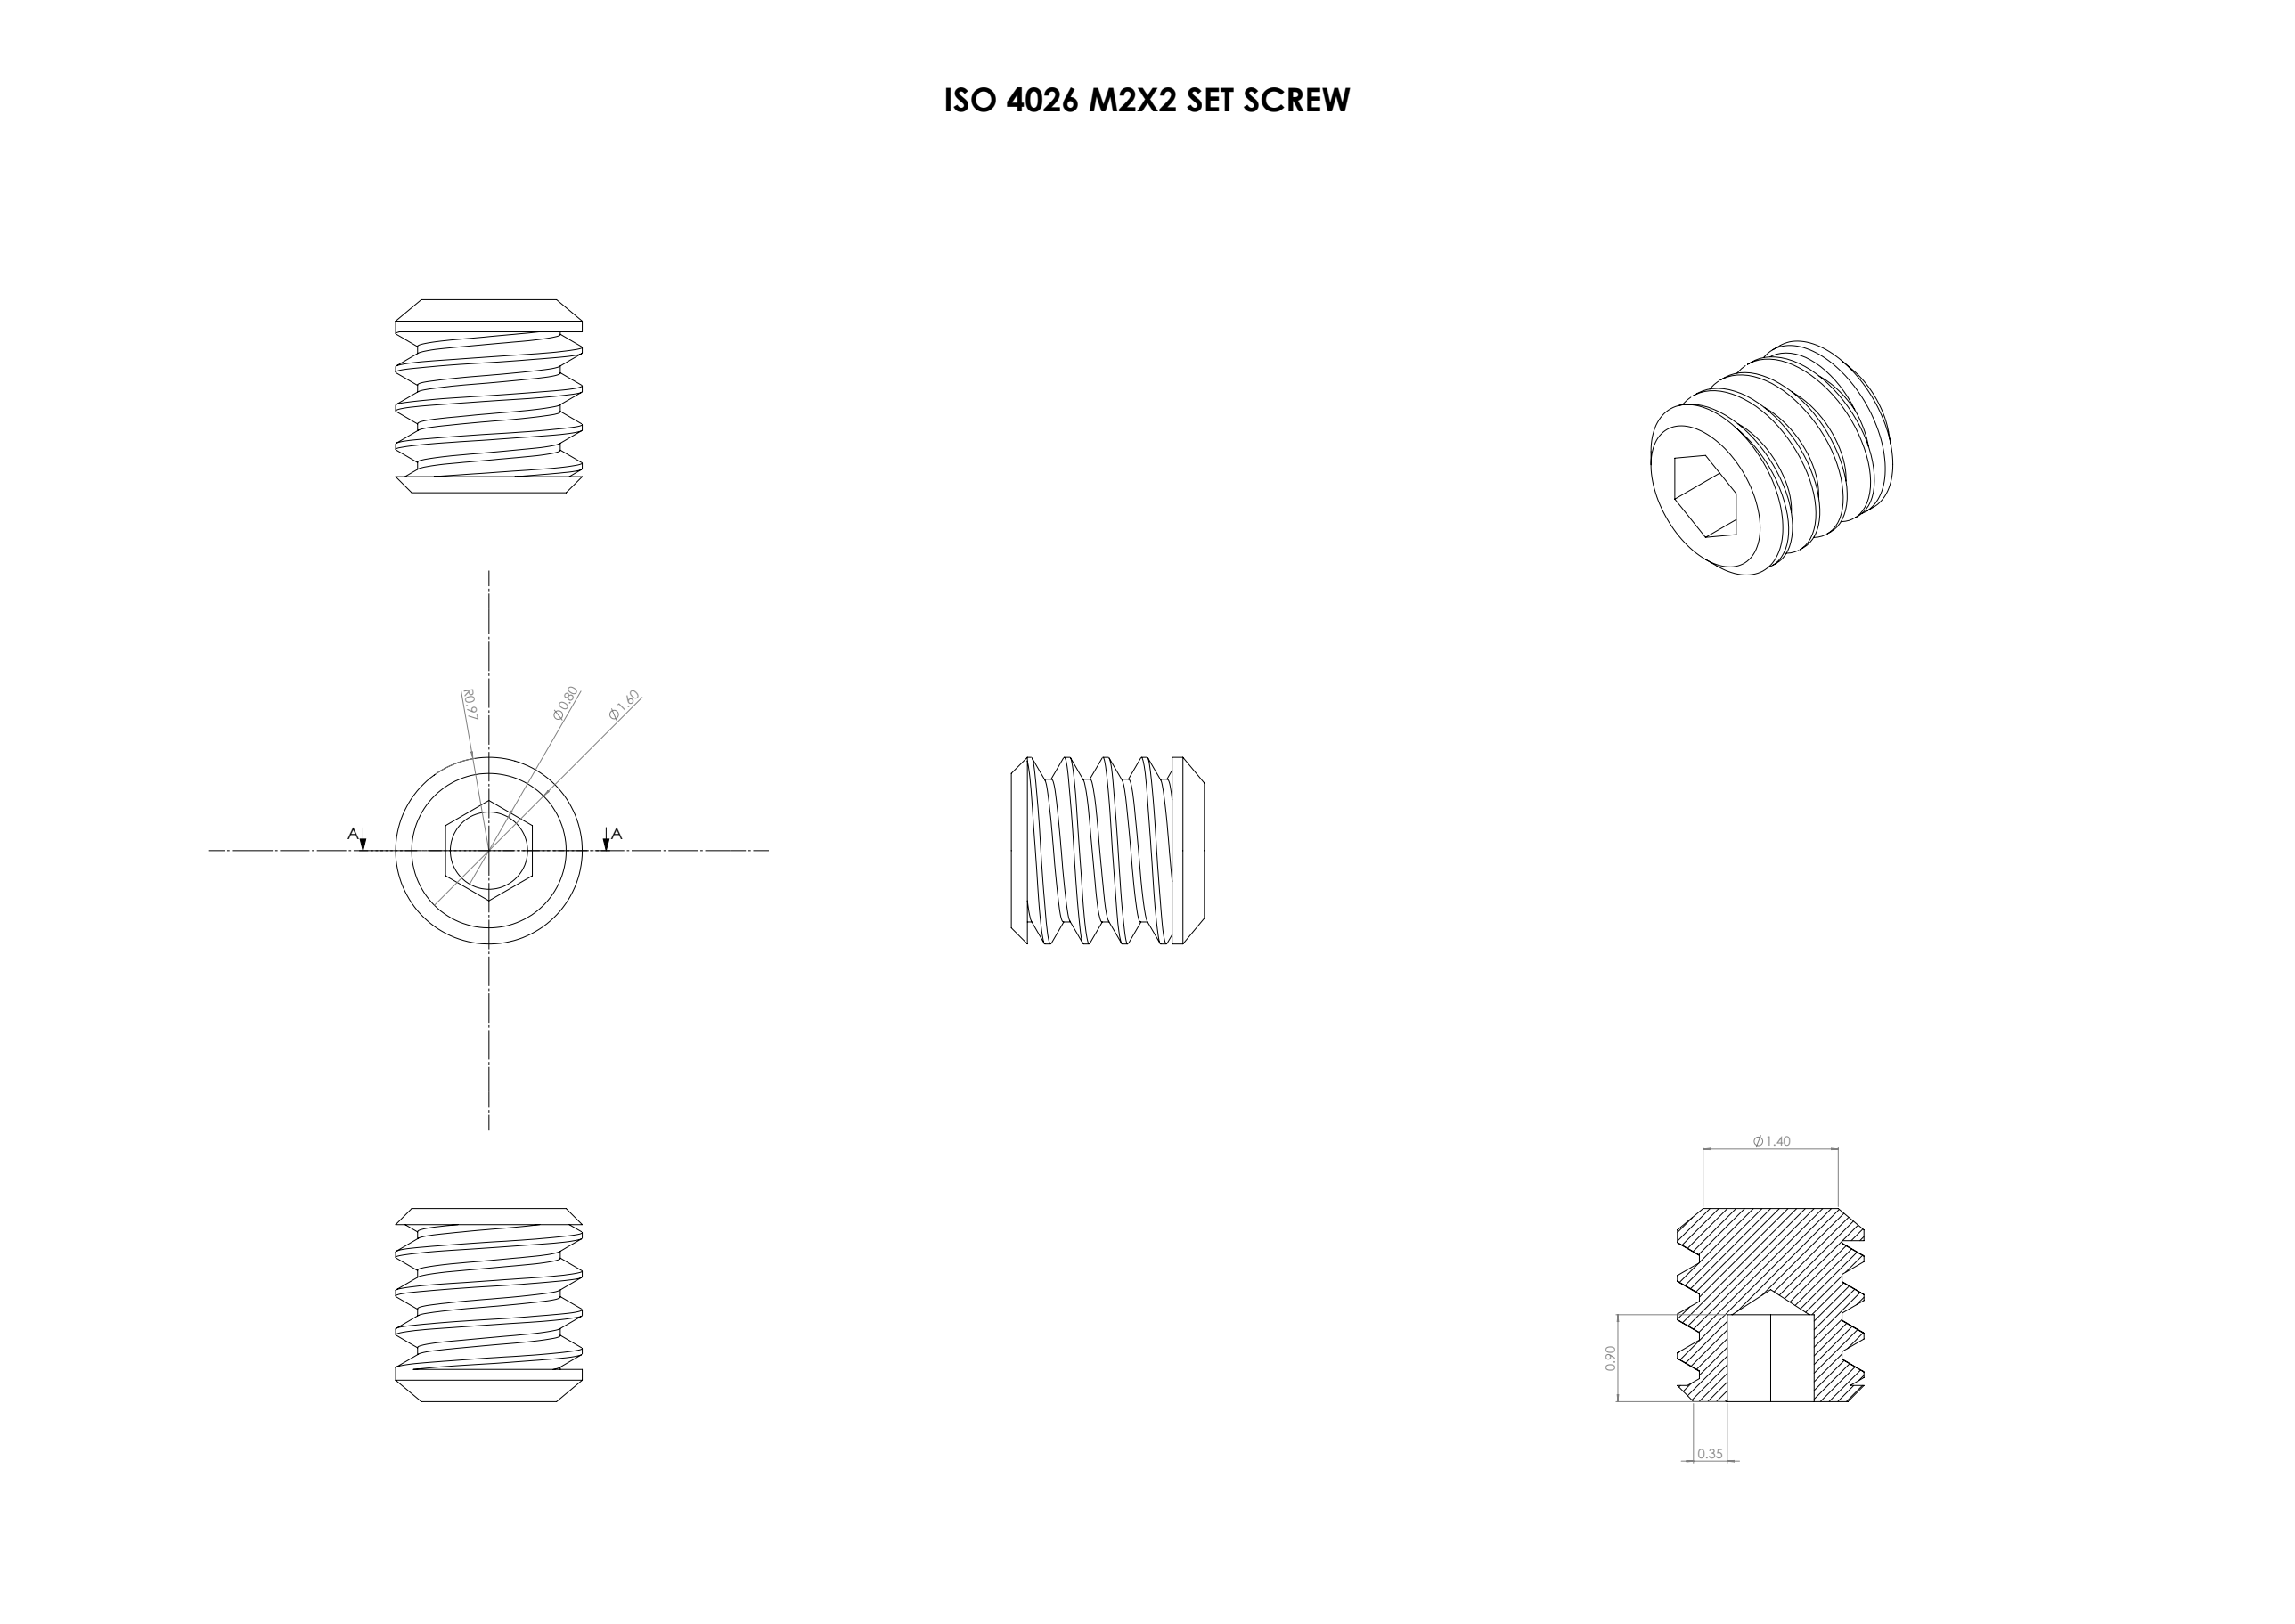
ISO-10303-21;
HEADER;
/* Generated by software containing ST-Developer
 * from STEP Tools, Inc. (www.steptools.com) 
 */

FILE_DESCRIPTION(
/* description */ (''),
/* implementation_level */ '2;1');

FILE_NAME(
/* name */ '20_ISO_4026_M2x2_Set_Screw.step',
/* time_stamp */ '2026-10-19T23:00:43-07:00',
/* author */ (''),
/* organization */ (''),
/* preprocessor_version */ 'ST-DEVELOPER v20.2',
/* originating_system */ 'Autodesk Translation Framework v15.15.0.0',
/* authorisation */ '');

FILE_SCHEMA (('AUTOMOTIVE_DESIGN { 1 0 10303 214 3 1 1 }'));
ENDSEC;

DATA;
#10=MECHANICAL_DESIGN_GEOMETRIC_PRESENTATION_REPRESENTATION('',(#1009),#55002);
#470=B_SPLINE_SURFACE_WITH_KNOTS('',3,3,((#38097,#38098,#38099,#38100,#38101,
#38102,#38103,#38104,#38105,#38106,#38107,#38108,#38109,#38110,#38111,#38112,
#38113,#38114,#38115,#38116,#38117,#38118,#38119,#38120,#38121,#38122,#38123,
#38124,#38125),(#38126,#38127,#38128,#38129,#38130,#38131,#38132,#38133,
#38134,#38135,#38136,#38137,#38138,#38139,#38140,#38141,#38142,#38143,#38144,
#38145,#38146,#38147,#38148,#38149,#38150,#38151,#38152,#38153,#38154),
(#38155,#38156,#38157,#38158,#38159,#38160,#38161,#38162,#38163,#38164,
#38165,#38166,#38167,#38168,#38169,#38170,#38171,#38172,#38173,#38174,#38175,
#38176,#38177,#38178,#38179,#38180,#38181,#38182,#38183),(#38184,#38185,
#38186,#38187,#38188,#38189,#38190,#38191,#38192,#38193,#38194,#38195,#38196,
#38197,#38198,#38199,#38200,#38201,#38202,#38203,#38204,#38205,#38206,#38207,
#38208,#38209,#38210,#38211,#38212)),.UNSPECIFIED.,.F.,.F.,.F.,(4,4),(4,
1,1,1,1,1,1,1,1,1,1,1,1,1,1,1,1,1,1,1,1,1,1,1,1,1,4),(0.,0.0262983047615875),
(10.0522207760382,11.0378903501899,12.0235599243416,13.0092294984934,13.9948990726451,
14.9805686467968,15.9662382209486,16.9519077951003,17.937577369252,18.9232469434038,
19.9089165175555,20.8945860917073,21.880255665859,22.8659252400107,23.8515948141625,
24.8372643883142,25.8229339624659,26.8086035366177,27.7942731107694,28.7799426849212,
29.7656122590729,30.7512818332246,31.7369514073764,32.7226209815281,33.7082905556798,
34.6939601298316,35.6796297039833),.UNSPECIFIED.);
#471=B_SPLINE_SURFACE_WITH_KNOTS('',3,3,((#38342,#38343,#38344,#38345,#38346,
#38347,#38348,#38349,#38350,#38351,#38352,#38353,#38354,#38355,#38356,#38357,
#38358,#38359,#38360,#38361,#38362,#38363,#38364,#38365,#38366,#38367,#38368,
#38369,#38370),(#38371,#38372,#38373,#38374,#38375,#38376,#38377,#38378,
#38379,#38380,#38381,#38382,#38383,#38384,#38385,#38386,#38387,#38388,#38389,
#38390,#38391,#38392,#38393,#38394,#38395,#38396,#38397,#38398,#38399),
(#38400,#38401,#38402,#38403,#38404,#38405,#38406,#38407,#38408,#38409,
#38410,#38411,#38412,#38413,#38414,#38415,#38416,#38417,#38418,#38419,#38420,
#38421,#38422,#38423,#38424,#38425,#38426,#38427,#38428),(#38429,#38430,
#38431,#38432,#38433,#38434,#38435,#38436,#38437,#38438,#38439,#38440,#38441,
#38442,#38443,#38444,#38445,#38446,#38447,#38448,#38449,#38450,#38451,#38452,
#38453,#38454,#38455,#38456,#38457)),.UNSPECIFIED.,.F.,.F.,.F.,(4,4),(4,
1,1,1,1,1,1,1,1,1,1,1,1,1,1,1,1,1,1,1,1,1,1,1,1,1,4),(0.,0.0262983047615875),
(13.3593226216143,14.3449921957661,15.3306617699178,16.3163313440695,17.3020009182213,
18.287670492373,19.2733400665247,20.2590096406765,21.2446792148282,22.23034878898,
23.2160183631317,24.2016879372834,25.1873575114352,26.1730270855869,27.1586966597386,
28.1443662338904,29.1300358080421,30.1157053821939,31.1013749563456,32.0870445304973,
33.0727141046491,34.0583836788008,35.0440532529525,36.0297228271043,37.015392401256,
38.0010619754078,38.9867315495595),.UNSPECIFIED.);
#505=B_SPLINE_CURVE_WITH_KNOTS('',3,(#37754,#37755,#37756,#37757,#37758,
#37759,#37760,#37761,#37762,#37763,#37764,#37765,#37766,#37767,#37768,#37769,
#37770,#37771,#37772,#37773,#37774,#37775),.UNSPECIFIED.,.F.,.F.,(4,3,3,
3,3,3,3,4),(-8.63182595351423,-7.8853565932139,-6.89968701906216,-5.91401744491043,
-4.92834787075869,-3.94267829660695,-2.95700872245521,-2.34864064633464),
 .UNSPECIFIED.);
#506=B_SPLINE_CURVE_WITH_KNOTS('',3,(#37780,#37781,#37782,#37783),
 .UNSPECIFIED.,.F.,.F.,(4,4),(-2.34864064633464,-2.06546402602172),
 .UNSPECIFIED.);
#507=B_SPLINE_CURVE_WITH_KNOTS('',3,(#37786,#37787,#37788,#37789,#37790,
#37791,#37792,#37793,#37794,#37795,#37796,#37797,#37798,#37799,#37800,#37801,
#37802,#37803,#37804),.UNSPECIFIED.,.F.,.F.,(4,3,3,3,3,3,4),(0.,0.985669574151735,
1.97133914830348,2.95700872245521,3.94267829660695,4.92834787075869,5.65574249191081),
 .UNSPECIFIED.);
#508=B_SPLINE_CURVE_WITH_KNOTS('',3,(#37809,#37810,#37811,#37812,#37813,
#37814,#37815,#37816,#37817,#37818,#37819,#37820,#37821,#37822,#37823,#37824,
#37825,#37826,#37827,#37828,#37829,#37830,#37831,#37832,#37833),
 .UNSPECIFIED.,.F.,.F.,(4,3,3,3,3,3,3,3,4),(-14.9150112606938,-14.7850436122761,
-13.7993740381243,-12.8137044639726,-11.8280348898208,-10.8423653156691,
-9.85669574151737,-8.87102616736564,-8.63182595351423),.UNSPECIFIED.);
#509=B_SPLINE_CURVE_WITH_KNOTS('',3,(#37834,#37835,#37836,#37837,#37838,
#37839,#37840,#37841,#37842,#37843,#37844,#37845,#37846,#37847,#37848,#37849,
#37850,#37851,#37852,#37853,#37854,#37855,#37856,#37857,#37858),
 .UNSPECIFIED.,.F.,.F.,(4,3,3,3,3,3,3,3,4),(5.65574249191081,5.91401744491043,
6.89968701906216,7.8853565932139,8.87102616736564,9.85669574151738,10.8423653156691,
11.8280348898208,11.9389277990904),.UNSPECIFIED.);
#510=B_SPLINE_CURVE_WITH_KNOTS('',3,(#37863,#37864,#37865,#37866,#37867,
#37868,#37869,#37870,#37871,#37872,#37873,#37874,#37875,#37876,#37877,#37878,
#37879,#37880,#37881,#37882,#37883,#37884),.UNSPECIFIED.,.F.,.F.,(4,3,3,
3,3,3,3,4),(-21.1981965678734,-20.6990610571865,-19.7133914830348,-18.727721908883,
-17.7420523347313,-16.7563827605795,-15.7707131864278,-14.9150112606938),
 .UNSPECIFIED.);
#511=B_SPLINE_CURVE_WITH_KNOTS('',3,(#37885,#37886,#37887,#37888,#37889,
#37890,#37891,#37892,#37893,#37894,#37895,#37896,#37897,#37898,#37899,#37900,
#37901,#37902,#37903,#37904,#37905,#37906),.UNSPECIFIED.,.F.,.F.,(4,3,3,
3,3,3,3,4),(11.9389277990904,12.8137044639726,13.7993740381243,14.7850436122761,
15.7707131864278,16.7563827605795,17.7420523347313,18.22211310627),
 .UNSPECIFIED.);
#512=B_SPLINE_CURVE_WITH_KNOTS('',3,(#37912,#37913,#37914,#37915,#37916,
#37917),.UNSPECIFIED.,.F.,.F.,(4,1,1,4),(34.5575191894877,35.0440532529525,
36.0297228271043,36.9212675235378),.UNSPECIFIED.);
#513=B_SPLINE_CURVE_WITH_KNOTS('',3,(#37920,#37921,#37922,#37923,#37924),
 .UNSPECIFIED.,.F.,.F.,(4,1,4),(34.5575191894877,34.6939601298316,35.6796297039833),
 .UNSPECIFIED.);
#514=B_SPLINE_CURVE_WITH_KNOTS('',3,(#37929,#37930,#37931,#37932,#37933,
#37934,#37935,#37936,#37937,#37938),.UNSPECIFIED.,.F.,.F.,(4,1,1,1,1,1,
1,4),(28.2743338823081,29.1300358080421,30.1157053821939,31.1013749563456,
32.0870445304973,33.0727141046491,34.0583836788008,34.5575191894877),
 .UNSPECIFIED.);
#515=B_SPLINE_CURVE_WITH_KNOTS('',3,(#37939,#37940,#37941,#37942,#37943,
#37944,#37945,#37946,#37947,#37948),.UNSPECIFIED.,.F.,.F.,(4,1,1,1,1,1,
1,4),(28.2743338823081,28.7799426849212,29.7656122590729,30.7512818332246,
31.7369514073764,32.7226209815281,33.7082905556798,34.5575191894877),
 .UNSPECIFIED.);
#516=B_SPLINE_CURVE_WITH_KNOTS('',3,(#37953,#37954,#37955,#37956,#37957,
#37958,#37959,#37960,#37961,#37962,#37963),.UNSPECIFIED.,.F.,.F.,(4,1,1,
1,1,1,1,1,4),(21.9911485751285,22.23034878898,23.2160183631317,24.2016879372834,
25.1873575114352,26.1730270855869,27.1586966597386,28.1443662338904,28.2743338823081),
 .UNSPECIFIED.);
#517=B_SPLINE_CURVE_WITH_KNOTS('',3,(#37964,#37965,#37966,#37967,#37968,
#37969,#37970,#37971,#37972,#37973),.UNSPECIFIED.,.F.,.F.,(4,1,1,1,1,1,
1,4),(21.9911485751285,22.8659252400107,23.8515948141625,24.8372643883142,
25.8229339624659,26.8086035366177,27.7942731107694,28.2743338823081),
 .UNSPECIFIED.);
#518=B_SPLINE_CURVE_WITH_KNOTS('',3,(#37978,#37979,#37980,#37981,#37982,
#37983,#37984,#37985,#37986,#37987),.UNSPECIFIED.,.F.,.F.,(4,1,1,1,1,1,
1,4),(15.707963267949,16.3163313440695,17.3020009182213,18.287670492373,
19.2733400665247,20.2590096406765,21.2446792148282,21.9911485751285),
 .UNSPECIFIED.);
#519=B_SPLINE_CURVE_WITH_KNOTS('',3,(#37988,#37989,#37990,#37991,#37992,
#37993,#37994,#37995,#37996,#37997,#37998),.UNSPECIFIED.,.F.,.F.,(4,1,1,
1,1,1,1,1,4),(15.707963267949,15.9662382209486,16.9519077951003,17.937577369252,
18.9232469434038,19.9089165175555,20.8945860917073,21.880255665859,21.9911485751285),
 .UNSPECIFIED.);
#520=B_SPLINE_CURVE_WITH_KNOTS('',3,(#38001,#38002,#38003,#38004,#38005,
#38006,#38007,#38008,#38009,#38010,#38011,#38012,#38013,#38014,#38015,#38016,
#38017,#38018,#38019,#38020,#38021,#38022,#38023,#38024,#38025,#38026,#38027,
#38028,#38029,#38030,#38031,#38032,#38033,#38034,#38035,#38036,#38037,#38038,
#38039,#38040,#38041,#38042,#38043,#38044,#38045,#38046),.UNSPECIFIED.,
 .F.,.F.,(4,3,3,3,3,3,3,3,3,3,3,3,3,3,3,4),(-0.178587760439503,-0.171463223481926,
-0.158469202239697,-0.149838461616654,-0.140115954947833,-0.131832290711792,
-0.111519735101834,-0.104220668242419,-0.0909951576576451,-0.0752259129616406,
-0.0672217662272291,-0.0504163246704218,-0.0371902256154733,-0.0290084673554581,
-0.00644509207244406,0.),.UNSPECIFIED.);
#521=B_SPLINE_CURVE_WITH_KNOTS('',3,(#38051,#38052,#38053,#38054,#38055,
#38056,#38057,#38058,#38059,#38060,#38061,#38062,#38063,#38064,#38065,#38066,
#38067,#38068,#38069,#38070,#38071,#38072,#38073,#38074,#38075,#38076,#38077,
#38078,#38079,#38080,#38081,#38082,#38083,#38084,#38085,#38086,#38087,#38088,
#38089,#38090,#38091,#38092,#38093,#38094,#38095,#38096),.UNSPECIFIED.,
 .F.,.F.,(4,3,3,3,3,3,3,3,3,3,3,3,3,3,3,4),(-0.177567088092161,-0.168491849215037,
-0.152129281927587,-0.143009688907872,-0.128326089911933,-0.120351006519644,
-0.0990535795520566,-0.087638613810708,-0.079080103543658,-0.064425434388532,
-0.0552021544374827,-0.041401615828112,-0.0308502855955504,-0.0238678565643904,
-0.00551137719623127,0.),.UNSPECIFIED.);
#522=B_SPLINE_CURVE_WITH_KNOTS('',3,(#38213,#38214,#38215,#38216,#38217,
#38218,#38219,#38220,#38221,#38222,#38223,#38224,#38225,#38226,#38227,#38228,
#38229,#38230,#38231),.UNSPECIFIED.,.F.,.F.,(4,3,3,3,3,3,4),(18.22211310627,
18.727721908883,19.7133914830347,20.6990610571865,21.6847306313382,22.67040020549,
23.5619449019235),.UNSPECIFIED.);
#523=B_SPLINE_CURVE_WITH_KNOTS('',3,(#38233,#38234,#38235,#38236,#38237,
#38238,#38239,#38240,#38241,#38242,#38243,#38244,#38245,#38246,#38247,#38248,
#38249,#38250,#38251,#38252,#38253,#38254,#38255,#38256,#38257,#38258,#38259,
#38260,#38261,#38262,#38263,#38264,#38265,#38266,#38267,#38268,#38269,#38270,
#38271,#38272,#38273,#38274,#38275,#38276,#38277,#38278),.UNSPECIFIED.,
 .F.,.F.,(4,3,3,3,3,3,3,3,3,3,3,3,3,3,3,4),(-0.178587760439501,-0.171463223481924,
-0.158469220396003,-0.149838461060004,-0.140115983264454,-0.131832291484538,
-0.11151973540878,-0.104220666177739,-0.0909951576576466,-0.0752259249257156,
-0.0672217660243099,-0.0504163245182324,-0.0371902270455756,-0.0290084696776603,
-0.00644510100322751,0.),.UNSPECIFIED.);
#524=B_SPLINE_CURVE_WITH_KNOTS('',3,(#38279,#38280,#38281,#38282,#38283,
#38284,#38285),.UNSPECIFIED.,.F.,.F.,(4,1,1,1,4),(12.1176848020599,13.0092294984934,
13.9948990726451,14.9805686467968,15.707963267949),.UNSPECIFIED.);
#525=B_SPLINE_CURVE_WITH_KNOTS('',3,(#38288,#38289,#38290,#38291,#38292,
#38293,#38294,#38295,#38296,#38297,#38298,#38299,#38300,#38301,#38302,#38303,
#38304,#38305,#38306,#38307,#38308,#38309,#38310,#38311,#38312,#38313,#38314,
#38315,#38316,#38317,#38318,#38319,#38320,#38321,#38322,#38323,#38324,#38325,
#38326,#38327,#38328,#38329,#38330,#38331,#38332,#38333),.UNSPECIFIED.,
 .F.,.F.,(4,3,3,3,3,3,3,3,3,3,3,3,3,3,3,4),(-0.177567088092159,-0.168491849215035,
-0.152129287596336,-0.143009693943577,-0.128326090026494,-0.120351011600958,
-0.0990535966185752,-0.087638608675612,-0.0790801035436585,-0.0644254494454798,
-0.0552021579381271,-0.0414016184535953,-0.0308502860822931,-0.0238678558967309,
-0.00551135674322404,0.),.UNSPECIFIED.);
#526=B_SPLINE_CURVE_WITH_KNOTS('',3,(#38336,#38337,#38338,#38339,#38340,
#38341),.UNSPECIFIED.,.F.,.F.,(4,1,1,4),(13.3593226216143,14.3449921957661,
15.3306617699178,15.707963267949),.UNSPECIFIED.);
#527=B_SPLINE_CURVE_WITH_KNOTS('',3,(#38458,#38459,#38460,#38461,#38462,
#38463,#38464,#38465,#38466,#38467,#38468,#38469,#38470,#38471,#38472,#38473),
 .UNSPECIFIED.,.F.,.F.,(4,3,3,3,3,4),(-25.6274089279452,-24.6417393537934,
-23.6560697796417,-22.67040020549,-21.6847306313382,-21.1981965678734),
 .UNSPECIFIED.);
#969=SHAPE_REPRESENTATION_RELATIONSHIP('SRR','None',#55117,#989);
#989=ADVANCED_BREP_SHAPE_REPRESENTATION('',(#1029),#54995);
#1009=STYLED_ITEM('',(#55393),#1029);
#1029=MANIFOLD_SOLID_BREP('Set Screw M2x2',#24542);
#1259=FACE_BOUND('',#4702,.T.);
#1260=FACE_BOUND('',#4707,.T.);
#1537=PLANE('',#26162);
#1538=PLANE('',#26165);
#1539=PLANE('',#26172);
#1540=PLANE('',#26173);
#1541=PLANE('',#26174);
#1542=PLANE('',#26175);
#1543=PLANE('',#26176);
#1544=PLANE('',#26177);
#1545=PLANE('',#26178);
#1546=PLANE('',#26179);
#1547=PLANE('',#26184);
#2193=CYLINDRICAL_SURFACE('',#26152,0.096675);
#2194=CYLINDRICAL_SURFACE('',#26155,0.096675);
#2195=CYLINDRICAL_SURFACE('',#26156,0.096675);
#2196=CYLINDRICAL_SURFACE('',#26157,0.0739);
#2197=CYLINDRICAL_SURFACE('',#26159,0.0739);
#2198=CYLINDRICAL_SURFACE('',#26160,0.0739);
#2199=CYLINDRICAL_SURFACE('',#26161,0.0739);
#2200=CYLINDRICAL_SURFACE('',#26167,0.0739);
#2201=CYLINDRICAL_SURFACE('',#26168,0.096675);
#3094=FACE_OUTER_BOUND('',#4681,.T.);
#3095=FACE_OUTER_BOUND('',#4682,.T.);
#3096=FACE_OUTER_BOUND('',#4683,.T.);
#3097=FACE_OUTER_BOUND('',#4684,.T.);
#3098=FACE_OUTER_BOUND('',#4685,.T.);
#3099=FACE_OUTER_BOUND('',#4686,.T.);
#3100=FACE_OUTER_BOUND('',#4687,.T.);
#3101=FACE_OUTER_BOUND('',#4688,.T.);
#3102=FACE_OUTER_BOUND('',#4689,.T.);
#3103=FACE_OUTER_BOUND('',#4690,.T.);
#3104=FACE_OUTER_BOUND('',#4691,.T.);
#3105=FACE_OUTER_BOUND('',#4692,.T.);
#3106=FACE_OUTER_BOUND('',#4693,.T.);
#3107=FACE_OUTER_BOUND('',#4694,.T.);
#3108=FACE_OUTER_BOUND('',#4695,.T.);
#3109=FACE_OUTER_BOUND('',#4696,.T.);
#3110=FACE_OUTER_BOUND('',#4697,.T.);
#3111=FACE_OUTER_BOUND('',#4698,.T.);
#3112=FACE_OUTER_BOUND('',#4699,.T.);
#3113=FACE_OUTER_BOUND('',#4700,.T.);
#3114=FACE_OUTER_BOUND('',#4701,.T.);
#3115=FACE_OUTER_BOUND('',#4703,.T.);
#3116=FACE_OUTER_BOUND('',#4704,.T.);
#3117=FACE_OUTER_BOUND('',#4705,.T.);
#3118=FACE_OUTER_BOUND('',#4706,.T.);
#4681=EDGE_LOOP('',(#19074,#19075,#19076,#19077,#19078,#19079,#19080,#19081));
#4682=EDGE_LOOP('',(#19082,#19083,#19084,#19085));
#4683=EDGE_LOOP('',(#19086,#19087,#19088,#19089));
#4684=EDGE_LOOP('',(#19090,#19091,#19092,#19093));
#4685=EDGE_LOOP('',(#19094,#19095,#19096,#19097));
#4686=EDGE_LOOP('',(#19098,#19099,#19100,#19101));
#4687=EDGE_LOOP('',(#19102,#19103,#19104,#19105));
#4688=EDGE_LOOP('',(#19106,#19107,#19108,#19109,#19110));
#4689=EDGE_LOOP('',(#19111,#19112,#19113,#19114,#19115,#19116,#19117,#19118,
#19119,#19120,#19121));
#4690=EDGE_LOOP('',(#19122,#19123,#19124,#19125));
#4691=EDGE_LOOP('',(#19126,#19127,#19128,#19129));
#4692=EDGE_LOOP('',(#19130,#19131,#19132,#19133,#19134,#19135,#19136,#19137,
#19138,#19139,#19140,#19141));
#4693=EDGE_LOOP('',(#19142,#19143,#19144,#19145));
#4694=EDGE_LOOP('',(#19146,#19147,#19148));
#4695=EDGE_LOOP('',(#19149,#19150,#19151,#19152));
#4696=EDGE_LOOP('',(#19153,#19154,#19155,#19156));
#4697=EDGE_LOOP('',(#19157,#19158,#19159,#19160));
#4698=EDGE_LOOP('',(#19161,#19162,#19163,#19164));
#4699=EDGE_LOOP('',(#19165,#19166,#19167,#19168));
#4700=EDGE_LOOP('',(#19169,#19170,#19171,#19172));
#4701=EDGE_LOOP('',(#19173,#19174,#19175,#19176,#19177,#19178));
#4702=EDGE_LOOP('',(#19179));
#4703=EDGE_LOOP('',(#19180));
#4704=EDGE_LOOP('',(#19181,#19182,#19183,#19184));
#4705=EDGE_LOOP('',(#19185,#19186,#19187,#19188,#19189,#19190));
#4706=EDGE_LOOP('',(#19191));
#4707=EDGE_LOOP('',(#19192,#19193,#19194,#19195,#19196,#19197));
#6265=LINE('',#37752,#8086);
#6266=LINE('',#37777,#8087);
#6267=LINE('',#37808,#8088);
#6268=LINE('',#37862,#8089);
#6269=LINE('',#37910,#8090);
#6270=LINE('',#37928,#8091);
#6271=LINE('',#37952,#8092);
#6272=LINE('',#37977,#8093);
#6273=LINE('',#38479,#8094);
#6274=LINE('',#38484,#8095);
#6275=LINE('',#38486,#8096);
#6276=LINE('',#38488,#8097);
#6277=LINE('',#38489,#8098);
#6278=LINE('',#38492,#8099);
#6279=LINE('',#38494,#8100);
#6280=LINE('',#38495,#8101);
#6281=LINE('',#38498,#8102);
#6282=LINE('',#38500,#8103);
#6283=LINE('',#38501,#8104);
#6284=LINE('',#38504,#8105);
#6285=LINE('',#38506,#8106);
#6286=LINE('',#38507,#8107);
#6287=LINE('',#38510,#8108);
#6288=LINE('',#38512,#8109);
#6289=LINE('',#38513,#8110);
#6290=LINE('',#38515,#8111);
#6291=LINE('',#38516,#8112);
#6292=LINE('',#38522,#8113);
#6293=LINE('',#38526,#8114);
#8086=VECTOR('',#30847,0.1);
#8087=VECTOR('',#30848,0.1);
#8088=VECTOR('',#30855,0.1);
#8089=VECTOR('',#30858,0.1);
#8090=VECTOR('',#30861,0.0739);
#8091=VECTOR('',#30866,0.0739);
#8092=VECTOR('',#30869,0.0739);
#8093=VECTOR('',#30872,0.0739);
#8094=VECTOR('',#30891,0.0207846096908265);
#8095=VECTOR('',#30896,1.);
#8096=VECTOR('',#30897,1.);
#8097=VECTOR('',#30898,1.);
#8098=VECTOR('',#30899,1.);
#8099=VECTOR('',#30902,1.);
#8100=VECTOR('',#30903,1.);
#8101=VECTOR('',#30904,1.);
#8102=VECTOR('',#30907,1.);
#8103=VECTOR('',#30908,1.);
#8104=VECTOR('',#30909,1.);
#8105=VECTOR('',#30912,1.);
#8106=VECTOR('',#30913,1.);
#8107=VECTOR('',#30914,1.);
#8108=VECTOR('',#30917,1.);
#8109=VECTOR('',#30918,1.);
#8110=VECTOR('',#30919,1.);
#8111=VECTOR('',#30922,1.);
#8112=VECTOR('',#30923,1.);
#8113=VECTOR('',#30932,0.085);
#8114=VECTOR('',#30937,0.09);
#9710=CIRCLE('',#26153,0.096675);
#9711=CIRCLE('',#26154,0.096675);
#9712=CIRCLE('',#26158,0.0739);
#9713=CIRCLE('',#26163,0.096675);
#9714=CIRCLE('',#26164,0.096675);
#9715=CIRCLE('',#26166,0.0739);
#9716=CIRCLE('',#26169,0.096675);
#9717=CIRCLE('',#26171,0.0400285208940887);
#9718=CIRCLE('',#26180,0.07);
#9719=CIRCLE('',#26183,0.08);
#11061=VERTEX_POINT('',#37750);
#11062=VERTEX_POINT('',#37751);
#11063=VERTEX_POINT('',#37753);
#11064=VERTEX_POINT('',#37776);
#11065=VERTEX_POINT('',#37779);
#11066=VERTEX_POINT('',#37784);
#11067=VERTEX_POINT('',#37806);
#11068=VERTEX_POINT('',#37807);
#11069=VERTEX_POINT('',#37860);
#11070=VERTEX_POINT('',#37861);
#11071=VERTEX_POINT('',#37908);
#11072=VERTEX_POINT('',#37909);
#11073=VERTEX_POINT('',#37911);
#11074=VERTEX_POINT('',#37918);
#11075=VERTEX_POINT('',#37926);
#11076=VERTEX_POINT('',#37927);
#11077=VERTEX_POINT('',#37950);
#11078=VERTEX_POINT('',#37951);
#11079=VERTEX_POINT('',#37975);
#11080=VERTEX_POINT('',#37976);
#11081=VERTEX_POINT('',#38000);
#11082=VERTEX_POINT('',#38047);
#11083=VERTEX_POINT('',#38049);
#11084=VERTEX_POINT('',#38232);
#11085=VERTEX_POINT('',#38287);
#11086=VERTEX_POINT('',#38477);
#11087=VERTEX_POINT('',#38478);
#11088=VERTEX_POINT('',#38482);
#11089=VERTEX_POINT('',#38483);
#11090=VERTEX_POINT('',#38485);
#11091=VERTEX_POINT('',#38487);
#11092=VERTEX_POINT('',#38491);
#11093=VERTEX_POINT('',#38493);
#11094=VERTEX_POINT('',#38497);
#11095=VERTEX_POINT('',#38499);
#11096=VERTEX_POINT('',#38503);
#11097=VERTEX_POINT('',#38505);
#11098=VERTEX_POINT('',#38509);
#11099=VERTEX_POINT('',#38511);
#11100=VERTEX_POINT('',#38519);
#11101=VERTEX_POINT('',#38524);
#13945=EDGE_CURVE('',#11061,#11062,#6265,.T.);
#13946=EDGE_CURVE('',#11061,#11063,#505,.T.);
#13947=EDGE_CURVE('',#11063,#11064,#6266,.T.);
#13948=EDGE_CURVE('',#11064,#11064,#9710,.T.);
#13949=EDGE_CURVE('',#11063,#11065,#506,.T.);
#13950=EDGE_CURVE('',#11065,#11066,#9711,.T.);
#13951=EDGE_CURVE('',#11066,#11062,#507,.T.);
#13952=EDGE_CURVE('',#11067,#11068,#6267,.T.);
#13953=EDGE_CURVE('',#11067,#11061,#508,.T.);
#13954=EDGE_CURVE('',#11062,#11068,#509,.T.);
#13955=EDGE_CURVE('',#11069,#11070,#6268,.T.);
#13956=EDGE_CURVE('',#11069,#11067,#510,.T.);
#13957=EDGE_CURVE('',#11068,#11070,#511,.T.);
#13958=EDGE_CURVE('',#11071,#11072,#6269,.T.);
#13959=EDGE_CURVE('',#11071,#11073,#512,.T.);
#13960=EDGE_CURVE('',#11074,#11073,#9712,.T.);
#13961=EDGE_CURVE('',#11072,#11074,#513,.T.);
#13962=EDGE_CURVE('',#11075,#11076,#6270,.T.);
#13963=EDGE_CURVE('',#11075,#11071,#514,.T.);
#13964=EDGE_CURVE('',#11076,#11072,#515,.T.);
#13965=EDGE_CURVE('',#11077,#11078,#6271,.T.);
#13966=EDGE_CURVE('',#11077,#11075,#516,.T.);
#13967=EDGE_CURVE('',#11078,#11076,#517,.T.);
#13968=EDGE_CURVE('',#11079,#11080,#6272,.T.);
#13969=EDGE_CURVE('',#11079,#11077,#518,.T.);
#13970=EDGE_CURVE('',#11080,#11078,#519,.T.);
#13971=EDGE_CURVE('',#11073,#11081,#520,.T.);
#13972=EDGE_CURVE('',#11082,#11081,#9713,.F.);
#13973=EDGE_CURVE('',#11083,#11082,#9714,.F.);
#13974=EDGE_CURVE('',#11083,#11074,#521,.T.);
#13975=EDGE_CURVE('',#11070,#11083,#522,.T.);
#13976=EDGE_CURVE('',#11084,#11066,#523,.T.);
#13977=EDGE_CURVE('',#11084,#11080,#524,.T.);
#13978=EDGE_CURVE('',#11065,#11085,#525,.T.);
#13979=EDGE_CURVE('',#11085,#11084,#9715,.T.);
#13980=EDGE_CURVE('',#11085,#11079,#526,.T.);
#13981=EDGE_CURVE('',#11081,#11069,#527,.T.);
#13982=EDGE_CURVE('',#11081,#11083,#9716,.F.);
#13983=EDGE_CURVE('',#11086,#11087,#6273,.T.);
#13984=EDGE_CURVE('',#11087,#11087,#9717,.T.);
#13985=EDGE_CURVE('',#11088,#11089,#6274,.T.);
#13986=EDGE_CURVE('',#11088,#11090,#6275,.T.);
#13987=EDGE_CURVE('',#11090,#11091,#6276,.T.);
#13988=EDGE_CURVE('',#11089,#11091,#6277,.T.);
#13989=EDGE_CURVE('',#11092,#11088,#6278,.T.);
#13990=EDGE_CURVE('',#11092,#11093,#6279,.T.);
#13991=EDGE_CURVE('',#11093,#11090,#6280,.T.);
#13992=EDGE_CURVE('',#11094,#11092,#6281,.T.);
#13993=EDGE_CURVE('',#11094,#11095,#6282,.T.);
#13994=EDGE_CURVE('',#11095,#11093,#6283,.T.);
#13995=EDGE_CURVE('',#11096,#11094,#6284,.T.);
#13996=EDGE_CURVE('',#11096,#11097,#6285,.T.);
#13997=EDGE_CURVE('',#11097,#11095,#6286,.T.);
#13998=EDGE_CURVE('',#11098,#11096,#6287,.T.);
#13999=EDGE_CURVE('',#11098,#11099,#6288,.T.);
#14000=EDGE_CURVE('',#11099,#11097,#6289,.T.);
#14001=EDGE_CURVE('',#11089,#11098,#6290,.T.);
#14002=EDGE_CURVE('',#11091,#11099,#6291,.T.);
#14003=EDGE_CURVE('',#11100,#11100,#9718,.T.);
#14004=EDGE_CURVE('',#11064,#11100,#6292,.T.);
#14005=EDGE_CURVE('',#11101,#11101,#9719,.T.);
#14006=EDGE_CURVE('',#11101,#11082,#6293,.T.);
#19074=ORIENTED_EDGE('',*,*,#13945,.F.);
#19075=ORIENTED_EDGE('',*,*,#13946,.T.);
#19076=ORIENTED_EDGE('',*,*,#13947,.T.);
#19077=ORIENTED_EDGE('',*,*,#13948,.T.);
#19078=ORIENTED_EDGE('',*,*,#13947,.F.);
#19079=ORIENTED_EDGE('',*,*,#13949,.T.);
#19080=ORIENTED_EDGE('',*,*,#13950,.T.);
#19081=ORIENTED_EDGE('',*,*,#13951,.T.);
#19082=ORIENTED_EDGE('',*,*,#13952,.F.);
#19083=ORIENTED_EDGE('',*,*,#13953,.T.);
#19084=ORIENTED_EDGE('',*,*,#13945,.T.);
#19085=ORIENTED_EDGE('',*,*,#13954,.T.);
#19086=ORIENTED_EDGE('',*,*,#13955,.F.);
#19087=ORIENTED_EDGE('',*,*,#13956,.T.);
#19088=ORIENTED_EDGE('',*,*,#13952,.T.);
#19089=ORIENTED_EDGE('',*,*,#13957,.T.);
#19090=ORIENTED_EDGE('',*,*,#13958,.F.);
#19091=ORIENTED_EDGE('',*,*,#13959,.T.);
#19092=ORIENTED_EDGE('',*,*,#13960,.F.);
#19093=ORIENTED_EDGE('',*,*,#13961,.F.);
#19094=ORIENTED_EDGE('',*,*,#13962,.F.);
#19095=ORIENTED_EDGE('',*,*,#13963,.T.);
#19096=ORIENTED_EDGE('',*,*,#13958,.T.);
#19097=ORIENTED_EDGE('',*,*,#13964,.F.);
#19098=ORIENTED_EDGE('',*,*,#13965,.F.);
#19099=ORIENTED_EDGE('',*,*,#13966,.T.);
#19100=ORIENTED_EDGE('',*,*,#13962,.T.);
#19101=ORIENTED_EDGE('',*,*,#13967,.F.);
#19102=ORIENTED_EDGE('',*,*,#13968,.F.);
#19103=ORIENTED_EDGE('',*,*,#13969,.T.);
#19104=ORIENTED_EDGE('',*,*,#13965,.T.);
#19105=ORIENTED_EDGE('',*,*,#13970,.F.);
#19106=ORIENTED_EDGE('',*,*,#13960,.T.);
#19107=ORIENTED_EDGE('',*,*,#13971,.T.);
#19108=ORIENTED_EDGE('',*,*,#13972,.F.);
#19109=ORIENTED_EDGE('',*,*,#13973,.F.);
#19110=ORIENTED_EDGE('',*,*,#13974,.T.);
#19111=ORIENTED_EDGE('',*,*,#13974,.F.);
#19112=ORIENTED_EDGE('',*,*,#13975,.F.);
#19113=ORIENTED_EDGE('',*,*,#13957,.F.);
#19114=ORIENTED_EDGE('',*,*,#13954,.F.);
#19115=ORIENTED_EDGE('',*,*,#13951,.F.);
#19116=ORIENTED_EDGE('',*,*,#13976,.F.);
#19117=ORIENTED_EDGE('',*,*,#13977,.T.);
#19118=ORIENTED_EDGE('',*,*,#13970,.T.);
#19119=ORIENTED_EDGE('',*,*,#13967,.T.);
#19120=ORIENTED_EDGE('',*,*,#13964,.T.);
#19121=ORIENTED_EDGE('',*,*,#13961,.T.);
#19122=ORIENTED_EDGE('',*,*,#13950,.F.);
#19123=ORIENTED_EDGE('',*,*,#13978,.T.);
#19124=ORIENTED_EDGE('',*,*,#13979,.T.);
#19125=ORIENTED_EDGE('',*,*,#13976,.T.);
#19126=ORIENTED_EDGE('',*,*,#13968,.T.);
#19127=ORIENTED_EDGE('',*,*,#13977,.F.);
#19128=ORIENTED_EDGE('',*,*,#13979,.F.);
#19129=ORIENTED_EDGE('',*,*,#13980,.T.);
#19130=ORIENTED_EDGE('',*,*,#13971,.F.);
#19131=ORIENTED_EDGE('',*,*,#13959,.F.);
#19132=ORIENTED_EDGE('',*,*,#13963,.F.);
#19133=ORIENTED_EDGE('',*,*,#13966,.F.);
#19134=ORIENTED_EDGE('',*,*,#13969,.F.);
#19135=ORIENTED_EDGE('',*,*,#13980,.F.);
#19136=ORIENTED_EDGE('',*,*,#13978,.F.);
#19137=ORIENTED_EDGE('',*,*,#13949,.F.);
#19138=ORIENTED_EDGE('',*,*,#13946,.F.);
#19139=ORIENTED_EDGE('',*,*,#13953,.F.);
#19140=ORIENTED_EDGE('',*,*,#13956,.F.);
#19141=ORIENTED_EDGE('',*,*,#13981,.F.);
#19142=ORIENTED_EDGE('',*,*,#13955,.T.);
#19143=ORIENTED_EDGE('',*,*,#13975,.T.);
#19144=ORIENTED_EDGE('',*,*,#13982,.F.);
#19145=ORIENTED_EDGE('',*,*,#13981,.T.);
#19146=ORIENTED_EDGE('',*,*,#13983,.T.);
#19147=ORIENTED_EDGE('',*,*,#13984,.F.);
#19148=ORIENTED_EDGE('',*,*,#13983,.F.);
#19149=ORIENTED_EDGE('',*,*,#13985,.F.);
#19150=ORIENTED_EDGE('',*,*,#13986,.T.);
#19151=ORIENTED_EDGE('',*,*,#13987,.T.);
#19152=ORIENTED_EDGE('',*,*,#13988,.F.);
#19153=ORIENTED_EDGE('',*,*,#13989,.F.);
#19154=ORIENTED_EDGE('',*,*,#13990,.T.);
#19155=ORIENTED_EDGE('',*,*,#13991,.T.);
#19156=ORIENTED_EDGE('',*,*,#13986,.F.);
#19157=ORIENTED_EDGE('',*,*,#13992,.F.);
#19158=ORIENTED_EDGE('',*,*,#13993,.T.);
#19159=ORIENTED_EDGE('',*,*,#13994,.T.);
#19160=ORIENTED_EDGE('',*,*,#13990,.F.);
#19161=ORIENTED_EDGE('',*,*,#13995,.F.);
#19162=ORIENTED_EDGE('',*,*,#13996,.T.);
#19163=ORIENTED_EDGE('',*,*,#13997,.T.);
#19164=ORIENTED_EDGE('',*,*,#13993,.F.);
#19165=ORIENTED_EDGE('',*,*,#13998,.F.);
#19166=ORIENTED_EDGE('',*,*,#13999,.T.);
#19167=ORIENTED_EDGE('',*,*,#14000,.T.);
#19168=ORIENTED_EDGE('',*,*,#13996,.F.);
#19169=ORIENTED_EDGE('',*,*,#14001,.F.);
#19170=ORIENTED_EDGE('',*,*,#13988,.T.);
#19171=ORIENTED_EDGE('',*,*,#14002,.T.);
#19172=ORIENTED_EDGE('',*,*,#13999,.F.);
#19173=ORIENTED_EDGE('',*,*,#14002,.F.);
#19174=ORIENTED_EDGE('',*,*,#13987,.F.);
#19175=ORIENTED_EDGE('',*,*,#13991,.F.);
#19176=ORIENTED_EDGE('',*,*,#13994,.F.);
#19177=ORIENTED_EDGE('',*,*,#13997,.F.);
#19178=ORIENTED_EDGE('',*,*,#14000,.F.);
#19179=ORIENTED_EDGE('',*,*,#13984,.T.);
#19180=ORIENTED_EDGE('',*,*,#14003,.F.);
#19181=ORIENTED_EDGE('',*,*,#13948,.F.);
#19182=ORIENTED_EDGE('',*,*,#14004,.T.);
#19183=ORIENTED_EDGE('',*,*,#14003,.T.);
#19184=ORIENTED_EDGE('',*,*,#14004,.F.);
#19185=ORIENTED_EDGE('',*,*,#14005,.F.);
#19186=ORIENTED_EDGE('',*,*,#14006,.T.);
#19187=ORIENTED_EDGE('',*,*,#13972,.T.);
#19188=ORIENTED_EDGE('',*,*,#13982,.T.);
#19189=ORIENTED_EDGE('',*,*,#13973,.T.);
#19190=ORIENTED_EDGE('',*,*,#14006,.F.);
#19191=ORIENTED_EDGE('',*,*,#14005,.T.);
#19192=ORIENTED_EDGE('',*,*,#13985,.T.);
#19193=ORIENTED_EDGE('',*,*,#14001,.T.);
#19194=ORIENTED_EDGE('',*,*,#13998,.T.);
#19195=ORIENTED_EDGE('',*,*,#13995,.T.);
#19196=ORIENTED_EDGE('',*,*,#13992,.T.);
#19197=ORIENTED_EDGE('',*,*,#13989,.T.);
#23131=CONICAL_SURFACE('',#26170,0.0207846096908265,0.995084829080935);
#23132=CONICAL_SURFACE('',#26181,0.085,0.876058050598194);
#23133=CONICAL_SURFACE('',#26182,0.09,0.785398163397448);
#23847=ADVANCED_FACE('',(#3094),#2193,.T.);
#23848=ADVANCED_FACE('',(#3095),#2194,.T.);
#23849=ADVANCED_FACE('',(#3096),#2195,.T.);
#23850=ADVANCED_FACE('',(#3097),#2196,.T.);
#23851=ADVANCED_FACE('',(#3098),#2197,.T.);
#23852=ADVANCED_FACE('',(#3099),#2198,.T.);
#23853=ADVANCED_FACE('',(#3100),#2199,.T.);
#23854=ADVANCED_FACE('',(#3101),#1537,.F.);
#23855=ADVANCED_FACE('',(#3102),#470,.F.);
#23856=ADVANCED_FACE('',(#3103),#1538,.T.);
#23857=ADVANCED_FACE('',(#3104),#2200,.T.);
#23858=ADVANCED_FACE('',(#3105),#471,.F.);
#23859=ADVANCED_FACE('',(#3106),#2201,.T.);
#23860=ADVANCED_FACE('',(#3107),#23131,.F.);
#23861=ADVANCED_FACE('',(#3108),#1539,.F.);
#23862=ADVANCED_FACE('',(#3109),#1540,.F.);
#23863=ADVANCED_FACE('',(#3110),#1541,.F.);
#23864=ADVANCED_FACE('',(#3111),#1542,.F.);
#23865=ADVANCED_FACE('',(#3112),#1543,.F.);
#23866=ADVANCED_FACE('',(#3113),#1544,.F.);
#23867=ADVANCED_FACE('',(#3114,#1259),#1545,.F.);
#23868=ADVANCED_FACE('',(#3115),#1546,.T.);
#23869=ADVANCED_FACE('',(#3116),#23132,.T.);
#23870=ADVANCED_FACE('',(#3117),#23133,.T.);
#23871=ADVANCED_FACE('',(#3118,#1260),#1547,.T.);
#24542=CLOSED_SHELL('',(#23847,#23848,#23849,#23850,#23851,#23852,#23853,
#23854,#23855,#23856,#23857,#23858,#23859,#23860,#23861,#23862,#23863,#23864,
#23865,#23866,#23867,#23868,#23869,#23870,#23871));
#26151=AXIS2_PLACEMENT_3D('',#37748,#30843,#30844);
#26152=AXIS2_PLACEMENT_3D('',#37749,#30845,#30846);
#26153=AXIS2_PLACEMENT_3D('',#37778,#30849,#30850);
#26154=AXIS2_PLACEMENT_3D('',#37785,#30851,#30852);
#26155=AXIS2_PLACEMENT_3D('',#37805,#30853,#30854);
#26156=AXIS2_PLACEMENT_3D('',#37859,#30856,#30857);
#26157=AXIS2_PLACEMENT_3D('',#37907,#30859,#30860);
#26158=AXIS2_PLACEMENT_3D('',#37919,#30862,#30863);
#26159=AXIS2_PLACEMENT_3D('',#37925,#30864,#30865);
#26160=AXIS2_PLACEMENT_3D('',#37949,#30867,#30868);
#26161=AXIS2_PLACEMENT_3D('',#37974,#30870,#30871);
#26162=AXIS2_PLACEMENT_3D('',#37999,#30873,#30874);
#26163=AXIS2_PLACEMENT_3D('',#38048,#30875,#30876);
#26164=AXIS2_PLACEMENT_3D('',#38050,#30877,#30878);
#26165=AXIS2_PLACEMENT_3D('',#38286,#30879,#30880);
#26166=AXIS2_PLACEMENT_3D('',#38334,#30881,#30882);
#26167=AXIS2_PLACEMENT_3D('',#38335,#30883,#30884);
#26168=AXIS2_PLACEMENT_3D('',#38474,#30885,#30886);
#26169=AXIS2_PLACEMENT_3D('',#38475,#30887,#30888);
#26170=AXIS2_PLACEMENT_3D('',#38476,#30889,#30890);
#26171=AXIS2_PLACEMENT_3D('',#38480,#30892,#30893);
#26172=AXIS2_PLACEMENT_3D('',#38481,#30894,#30895);
#26173=AXIS2_PLACEMENT_3D('',#38490,#30900,#30901);
#26174=AXIS2_PLACEMENT_3D('',#38496,#30905,#30906);
#26175=AXIS2_PLACEMENT_3D('',#38502,#30910,#30911);
#26176=AXIS2_PLACEMENT_3D('',#38508,#30915,#30916);
#26177=AXIS2_PLACEMENT_3D('',#38514,#30920,#30921);
#26178=AXIS2_PLACEMENT_3D('',#38517,#30924,#30925);
#26179=AXIS2_PLACEMENT_3D('',#38518,#30926,#30927);
#26180=AXIS2_PLACEMENT_3D('',#38520,#30928,#30929);
#26181=AXIS2_PLACEMENT_3D('',#38521,#30930,#30931);
#26182=AXIS2_PLACEMENT_3D('',#38523,#30933,#30934);
#26183=AXIS2_PLACEMENT_3D('',#38525,#30935,#30936);
#26184=AXIS2_PLACEMENT_3D('',#38527,#30938,#30939);
#30843=DIRECTION('axis',(0.,0.,1.));
#30844=DIRECTION('refdir',(1.,0.,0.));
#30845=DIRECTION('center_axis',(0.,0.,1.));
#30846=DIRECTION('ref_axis',(1.,0.,0.));
#30847=DIRECTION('',(0.,0.,-1.));
#30848=DIRECTION('',(0.,0.,-1.));
#30849=DIRECTION('center_axis',(0.,0.,1.));
#30850=DIRECTION('ref_axis',(1.,0.,0.));
#30851=DIRECTION('center_axis',(0.,0.,-1.));
#30852=DIRECTION('ref_axis',(1.,0.,0.));
#30853=DIRECTION('center_axis',(0.,0.,1.));
#30854=DIRECTION('ref_axis',(1.,0.,0.));
#30855=DIRECTION('',(0.,0.,-1.));
#30856=DIRECTION('center_axis',(0.,0.,1.));
#30857=DIRECTION('ref_axis',(1.,0.,0.));
#30858=DIRECTION('',(0.,0.,-1.));
#30859=DIRECTION('center_axis',(0.,0.,1.));
#30860=DIRECTION('ref_axis',(1.,7.2918327227141E-15,9.38957226509774E-17));
#30861=DIRECTION('',(0.,0.,1.));
#30862=DIRECTION('center_axis',(0.,0.,1.));
#30863=DIRECTION('ref_axis',(1.,7.2918327227141E-15,9.38957226509774E-17));
#30864=DIRECTION('center_axis',(0.,0.,1.));
#30865=DIRECTION('ref_axis',(1.,7.2918327227141E-15,9.38957226509774E-17));
#30866=DIRECTION('',(0.,0.,1.));
#30867=DIRECTION('center_axis',(0.,0.,1.));
#30868=DIRECTION('ref_axis',(1.,7.2918327227141E-15,9.38957226509774E-17));
#30869=DIRECTION('',(0.,0.,1.));
#30870=DIRECTION('center_axis',(0.,0.,1.));
#30871=DIRECTION('ref_axis',(1.,7.2918327227141E-15,9.38957226509774E-17));
#30872=DIRECTION('',(0.,0.,1.));
#30873=DIRECTION('center_axis',(0.,0.,1.));
#30874=DIRECTION('ref_axis',(1.,0.,0.));
#30875=DIRECTION('center_axis',(0.,0.,-1.));
#30876=DIRECTION('ref_axis',(1.,0.,0.));
#30877=DIRECTION('center_axis',(0.,0.,-1.));
#30878=DIRECTION('ref_axis',(1.,0.,0.));
#30879=DIRECTION('center_axis',(0.,0.,1.));
#30880=DIRECTION('ref_axis',(1.,0.,0.));
#30881=DIRECTION('center_axis',(0.,0.,-1.));
#30882=DIRECTION('ref_axis',(1.,7.2918327227141E-15,9.38957226509774E-17));
#30883=DIRECTION('center_axis',(0.,0.,1.));
#30884=DIRECTION('ref_axis',(0.222268344484715,0.974985529656735,9.38957226509774E-17));
#30885=DIRECTION('center_axis',(0.,0.,1.));
#30886=DIRECTION('ref_axis',(0.890895128280542,-0.454209060242083,0.));
#30887=DIRECTION('center_axis',(0.,0.,-1.));
#30888=DIRECTION('ref_axis',(1.,0.,0.));
#30889=DIRECTION('center_axis',(0.,0.,1.));
#30890=DIRECTION('ref_axis',(1.,0.,0.));
#30891=DIRECTION('',(-0.838805152831226,-1.02724004552307E-16,0.544431736385548));
#30892=DIRECTION('center_axis',(0.,0.,-1.));
#30893=DIRECTION('ref_axis',(1.,0.,0.));
#30894=DIRECTION('center_axis',(0.5,0.866025403784439,0.));
#30895=DIRECTION('ref_axis',(0.866025403784439,-0.5,0.));
#30896=DIRECTION('',(0.866025403784439,-0.5,0.));
#30897=DIRECTION('',(0.,0.,-1.));
#30898=DIRECTION('',(0.866025403784439,-0.5,0.));
#30899=DIRECTION('',(0.,0.,-1.));
#30900=DIRECTION('center_axis',(-0.5,0.866025403784439,0.));
#30901=DIRECTION('ref_axis',(0.866025403784439,0.5,0.));
#30902=DIRECTION('',(0.866025403784439,0.5,0.));
#30903=DIRECTION('',(0.,0.,-1.));
#30904=DIRECTION('',(0.866025403784439,0.5,0.));
#30905=DIRECTION('center_axis',(-1.,-1.33539075443303E-16,0.));
#30906=DIRECTION('ref_axis',(-1.33539075443303E-16,1.,0.));
#30907=DIRECTION('',(-1.33539075443303E-16,1.,0.));
#30908=DIRECTION('',(0.,0.,-1.));
#30909=DIRECTION('',(-1.33539075443303E-16,1.,0.));
#30910=DIRECTION('center_axis',(-0.5,-0.866025403784439,0.));
#30911=DIRECTION('ref_axis',(-0.866025403784439,0.5,0.));
#30912=DIRECTION('',(-0.866025403784439,0.5,0.));
#30913=DIRECTION('',(0.,0.,-1.));
#30914=DIRECTION('',(-0.866025403784439,0.5,0.));
#30915=DIRECTION('center_axis',(0.5,-0.866025403784439,0.));
#30916=DIRECTION('ref_axis',(-0.866025403784439,-0.5,0.));
#30917=DIRECTION('',(-0.866025403784439,-0.5,0.));
#30918=DIRECTION('',(0.,0.,-1.));
#30919=DIRECTION('',(-0.866025403784439,-0.5,0.));
#30920=DIRECTION('center_axis',(1.,-2.67078150886606E-16,0.));
#30921=DIRECTION('ref_axis',(-2.67078150886606E-16,-1.,0.));
#30922=DIRECTION('',(-2.67078150886606E-16,-1.,0.));
#30923=DIRECTION('',(-2.67078150886606E-16,-1.,0.));
#30924=DIRECTION('center_axis',(0.,0.,-1.));
#30925=DIRECTION('ref_axis',(-1.,0.,0.));
#30926=DIRECTION('center_axis',(0.,0.,-1.));
#30927=DIRECTION('ref_axis',(-1.,0.,0.));
#30928=DIRECTION('center_axis',(0.,0.,1.));
#30929=DIRECTION('ref_axis',(1.,0.,0.));
#30930=DIRECTION('center_axis',(0.,0.,1.));
#30931=DIRECTION('ref_axis',(1.,0.,0.));
#30932=DIRECTION('',(0.768221279597376,9.4079973109581E-17,-0.64018439966448));
#30933=DIRECTION('center_axis',(0.,0.,-1.));
#30934=DIRECTION('ref_axis',(1.,0.,0.));
#30935=DIRECTION('center_axis',(0.,0.,1.));
#30936=DIRECTION('ref_axis',(1.,0.,0.));
#30937=DIRECTION('',(-0.707106781186547,-8.65956056235493E-17,-0.707106781186548));
#30938=DIRECTION('center_axis',(0.,0.,1.));
#30939=DIRECTION('ref_axis',(1.,0.,0.));
#37748=CARTESIAN_POINT('',(0.,0.,0.));
#37749=CARTESIAN_POINT('Origin',(0.,0.,0.1025));
#37750=CARTESIAN_POINT('',(-0.0966658713741579,-8.30033664664526E-5,0.0751277583556343));
#37751=CARTESIAN_POINT('',(-0.0966485063039693,-8.22854894029733E-5,0.0693305749776991));
#37752=CARTESIAN_POINT('',(-0.096675,-1.1839272930757E-17,0.1025));
#37753=CARTESIAN_POINT('',(-0.0965779349718935,5.35477908776769E-5,0.0351277583556343));
#37754=CARTESIAN_POINT('Ctrl Pts',(-0.0966658713741579,-8.30033664664526E-5,
0.0751277583556343));
#37755=CARTESIAN_POINT('Ctrl Pts',(-0.0964554816322757,0.0239708948875215,
0.0735437011748551));
#37756=CARTESIAN_POINT('Ctrl Pts',(-0.0873429088905798,0.048167382154486,
0.0719596439940758));
#37757=CARTESIAN_POINT('Ctrl Pts',(-0.071078953014767,0.0657492986486455,
0.0703755868132966));
#37758=CARTESIAN_POINT('Ctrl Pts',(-0.0496033408668211,0.0889652014910574,
0.0682839310135428));
#37759=CARTESIAN_POINT('Ctrl Pts',(-0.015658810541703,0.100648154665348,
0.0661922752137891));
#37760=CARTESIAN_POINT('Ctrl Pts',(0.0155551384254827,0.0955677385731121,
0.0641006194140353));
#37761=CARTESIAN_POINT('Ctrl Pts',(0.0467690873926682,0.0904873224808759,
0.0620089636142815));
#37762=CARTESIAN_POINT('Ctrl Pts',(0.0752524550019215,0.0686435371221129,
0.0599173078145278));
#37763=CARTESIAN_POINT('Ctrl Pts',(0.0882585289492488,0.0398157711278956,
0.057825652014774));
#37764=CARTESIAN_POINT('Ctrl Pts',(0.101264602896576,0.010988005133678,
0.0557339962150202));
#37765=CARTESIAN_POINT('Ctrl Pts',(0.0987933831819777,-0.024823741495994,
0.0536423404152665));
#37766=CARTESIAN_POINT('Ctrl Pts',(0.0819414258178345,-0.0515867990200962,
0.0515506846155127));
#37767=CARTESIAN_POINT('Ctrl Pts',(0.0650894684536913,-0.0783498565441982,
0.049459028815759));
#37768=CARTESIAN_POINT('Ctrl Pts',(0.0338567734400037,-0.0960642249627305,
0.0473673730160052));
#37769=CARTESIAN_POINT('Ctrl Pts',(0.00224472816243995,-0.0967991363303525,
0.0452757172162514));
#37770=CARTESIAN_POINT('Ctrl Pts',(-0.0293673171151238,-0.0975340476979745,
0.0431840614164977));
#37771=CARTESIAN_POINT('Ctrl Pts',(-0.0613587126565637,-0.0812895020146863,
0.0410924056167439));
#37772=CARTESIAN_POINT('Ctrl Pts',(-0.079442849947587,-0.0553384044193135,
0.0390007498169901));
#37773=CARTESIAN_POINT('Ctrl Pts',(-0.0906046146003188,-0.0393210495862792,
0.0377097526632049));
#37774=CARTESIAN_POINT('Ctrl Pts',(-0.096468382952661,-0.0196059654673,
0.0364187555094196));
#37775=CARTESIAN_POINT('Ctrl Pts',(-0.0965779349718935,5.35477908776769E-5,
0.0351277583556343));
#37776=CARTESIAN_POINT('',(-0.096675,-1.1839272930757E-17,0.0222291666666667));
#37777=CARTESIAN_POINT('',(-0.096675,-1.1839272930757E-17,0.1025));
#37778=CARTESIAN_POINT('Origin',(0.,0.,0.0222291666666667));
#37779=CARTESIAN_POINT('',(-0.0929420004886496,0.02708977403664,0.033325));
#37780=CARTESIAN_POINT('Ctrl Pts',(-0.0965779349718935,5.35477908776769E-5,
0.0351277583556343));
#37781=CARTESIAN_POINT('Ctrl Pts',(-0.0966289280659962,0.00920444630111537,
0.0345268389037562));
#37782=CARTESIAN_POINT('Ctrl Pts',(-0.095433203415953,0.0183433047394809,
0.0339259194518781));
#37783=CARTESIAN_POINT('Ctrl Pts',(-0.0929447515460691,0.0270916053744145,
0.033325));
#37784=CARTESIAN_POINT('',(-0.0782614497120755,-0.0567556262758529,0.033325));
#37785=CARTESIAN_POINT('Origin',(0.,0.,0.033325));
#37786=CARTESIAN_POINT('Ctrl Pts',(-0.0782614497120756,-0.0567556262758528,
0.033325));
#37787=CARTESIAN_POINT('Ctrl Pts',(-0.0596140183847306,-0.0824689362125857,
0.0354166557997537));
#37788=CARTESIAN_POINT('Ctrl Pts',(-0.0274771552068993,-0.0980768870368331,
0.0375083115995075));
#37789=CARTESIAN_POINT('Ctrl Pts',(0.00406898269203012,-0.0967332918525559,
0.0395999673992613));
#37790=CARTESIAN_POINT('Ctrl Pts',(0.0356151205909597,-0.0953896966682786,
0.041691623199015));
#37791=CARTESIAN_POINT('Ctrl Pts',(0.0665705332109873,-0.0770945554754765,
0.0437832789987688));
#37792=CARTESIAN_POINT('Ctrl Pts',(0.0829257401395832,-0.0500177063557517,
0.0458749347985226));
#37793=CARTESIAN_POINT('Ctrl Pts',(0.0992809470681791,-0.022940857236027,
0.0479665905982763));
#37794=CARTESIAN_POINT('Ctrl Pts',(0.101035948305343,0.0129176998106204,
0.0500582463980301));
#37795=CARTESIAN_POINT('Ctrl Pts',(0.0874745068942844,0.0414936169721777,
0.0521499021977838));
#37796=CARTESIAN_POINT('Ctrl Pts',(0.0739130654832254,0.0700695341337352,
0.0542415579975376));
#37797=CARTESIAN_POINT('Ctrl Pts',(0.0450351814239432,0.0913628114102026,
0.0563332137972914));
#37798=CARTESIAN_POINT('Ctrl Pts',(0.0137340407189411,0.0958461699181061,
0.0584248695970452));
#37799=CARTESIAN_POINT('Ctrl Pts',(-0.0175670999860608,0.10032952842601,
0.0605165253967989));
#37800=CARTESIAN_POINT('Ctrl Pts',(-0.0512914973367827,0.0880029681653493,
0.0626081811965526));
#37801=CARTESIAN_POINT('Ctrl Pts',(-0.072322500665143,0.064382075719902,
0.0646998369963064));
#37802=CARTESIAN_POINT('Ctrl Pts',(-0.0878427511625237,0.0469505646311909,
0.0662434163234373));
#37803=CARTESIAN_POINT('Ctrl Pts',(-0.096450181952939,0.0233681626171319,
0.0677869956505682));
#37804=CARTESIAN_POINT('Ctrl Pts',(-0.0966485063039693,-8.22854894029733E-5,
0.0693305749776991));
#37805=CARTESIAN_POINT('Origin',(0.,0.,0.1025));
#37806=CARTESIAN_POINT('',(-0.0967646650617208,6.3821447323616E-5,0.115127758355634));
#37807=CARTESIAN_POINT('',(-0.0967793169573732,5.66163319584007E-5,0.109330574977699));
#37808=CARTESIAN_POINT('',(-0.096675,-1.1839272930757E-17,0.1025));
#37809=CARTESIAN_POINT('Ctrl Pts',(-0.0967646650617208,6.3821447323616E-5,
0.115127758355634));
#37810=CARTESIAN_POINT('Ctrl Pts',(-0.0967967436437804,0.00424079196011727,
0.114851958439798));
#37811=CARTESIAN_POINT('Ctrl Pts',(-0.0965491014611655,0.00841393489638481,
0.114576158523962));
#37812=CARTESIAN_POINT('Ctrl Pts',(-0.0960086603335039,0.012548805287274,
0.114300358608126));
#37813=CARTESIAN_POINT('Ctrl Pts',(-0.091909975909792,0.0439075009856079,
0.112208702808372));
#37814=CARTESIAN_POINT('Ctrl Pts',(-0.0709705314650557,0.0730648952004004,
0.110117047008618));
#37815=CARTESIAN_POINT('Ctrl Pts',(-0.042564880047698,0.0869675511134677,
0.108025391208864));
#37816=CARTESIAN_POINT('Ctrl Pts',(-0.0141592286303404,0.100870207026535,
0.105933735409111));
#37817=CARTESIAN_POINT('Ctrl Pts',(0.0217126297596384,0.0995181246378772,
0.103842079609357));
#37818=CARTESIAN_POINT('Ctrl Pts',(0.0489910406446355,0.0835165288481682,
0.101750423809603));
#37819=CARTESIAN_POINT('Ctrl Pts',(0.0762694515296325,0.0675149330584592,
0.0996587680098494));
#37820=CARTESIAN_POINT('Ctrl Pts',(0.0949544149096479,0.0368638238676987,
0.0975671122100956));
#37821=CARTESIAN_POINT('Ctrl Pts',(0.0966808481865763,0.0052855987430675,
0.0954754564103418));
#37822=CARTESIAN_POINT('Ctrl Pts',(0.0984072814635047,-0.0262926263815637,
0.093383800610588));
#37823=CARTESIAN_POINT('Ctrl Pts',(0.0831751846373464,-0.0587979674400657,
0.0912921448108343));
#37824=CARTESIAN_POINT('Ctrl Pts',(0.0578036983412537,-0.0776779752004735,
0.0892004890110805));
#37825=CARTESIAN_POINT('Ctrl Pts',(0.0324322120451609,-0.0965579829608814,
0.0871088332113267));
#37826=CARTESIAN_POINT('Ctrl Pts',(-0.00307866372086639,-0.101812657423195,
0.085017177411573));
#37827=CARTESIAN_POINT('Ctrl Pts',(-0.0328305038734412,-0.091089490875905,
0.0829255216118192));
#37828=CARTESIAN_POINT('Ctrl Pts',(-0.0625823440260158,-0.0803663243286154,
0.0808338658120654));
#37829=CARTESIAN_POINT('Ctrl Pts',(-0.086575148565138,-0.0536653167717232,
0.0787422100123117));
#37830=CARTESIAN_POINT('Ctrl Pts',(-0.0940682038493122,-0.0229403867380109,
0.0766505542125579));
#37831=CARTESIAN_POINT('Ctrl Pts',(-0.0958866027056606,-0.0154841255046677,
0.0761429555935834));
#37832=CARTESIAN_POINT('Ctrl Pts',(-0.0967332891061196,-0.00779088517959144,
0.0756353569746089));
#37833=CARTESIAN_POINT('Ctrl Pts',(-0.0966658713741579,-8.30033664664526E-5,
0.0751277583556343));
#37834=CARTESIAN_POINT('Ctrl Pts',(-0.0966485063039693,-8.22854894029733E-5,
0.0693305749776991));
#37835=CARTESIAN_POINT('Ctrl Pts',(-0.0967189250436074,-0.0084088020822012,
0.069878651450322));
#37836=CARTESIAN_POINT('Ctrl Pts',(-0.0957291768326631,-0.0167186827609739,
0.0704267279229449));
#37837=CARTESIAN_POINT('Ctrl Pts',(-0.0936122806995565,-0.0247306772532468,
0.0709748043955678));
#37838=CARTESIAN_POINT('Ctrl Pts',(-0.085533448099611,-0.0553073131507138,
0.0730664601953215));
#37839=CARTESIAN_POINT('Ctrl Pts',(-0.0610381735937214,-0.0815453603154133,
0.0751581159950752));
#37840=CARTESIAN_POINT('Ctrl Pts',(-0.0310877945671743,-0.0916989920757568,
0.0772497717948289));
#37841=CARTESIAN_POINT('Ctrl Pts',(-0.0011374155406272,-0.1018526238361,
0.0793414275945827));
#37842=CARTESIAN_POINT('Ctrl Pts',(0.0342680680065774,-0.0959218401920879,
0.0814330833943366));
#37843=CARTESIAN_POINT('Ctrl Pts',(0.0592751346151767,-0.0765613965401887,
0.0835247391940904));
#37844=CARTESIAN_POINT('Ctrl Pts',(0.0842822012237761,-0.0572009528882895,
0.0856163949938442));
#37845=CARTESIAN_POINT('Ctrl Pts',(0.0988908508937702,-0.0244108492285036,
0.0877080507935979));
#37846=CARTESIAN_POINT('Ctrl Pts',(0.096562264665659,0.00712872955992228,
0.0897997065933517));
#37847=CARTESIAN_POINT('Ctrl Pts',(0.0942336784375477,0.0386683083483482,
0.0918913623931054));
#37848=CARTESIAN_POINT('Ctrl Pts',(0.0749678563113312,0.0689573622654141,
0.0939830181928592));
#37849=CARTESIAN_POINT('Ctrl Pts',(0.047389275909168,0.0844357455165206,
0.096074673992613));
#37850=CARTESIAN_POINT('Ctrl Pts',(0.019810695507005,0.099914128767627,
0.0981663297923668));
#37851=CARTESIAN_POINT('Ctrl Pts',(-0.0160806431711048,0.100581841352774,
0.10025798559212));
#37852=CARTESIAN_POINT('Ctrl Pts',(-0.0442159874082662,0.0861399043308145,
0.102349641391874));
#37853=CARTESIAN_POINT('Ctrl Pts',(-0.0723513316454278,0.0716979673088548,
0.104441297191628));
#37854=CARTESIAN_POINT('Ctrl Pts',(-0.092730681441641,0.0421463806797884,
0.106532952991382));
#37855=CARTESIAN_POINT('Ctrl Pts',(-0.0962304983171589,0.0107152449419454,
0.108624608791136));
#37856=CARTESIAN_POINT('Ctrl Pts',(-0.0966242457609418,0.0071790801104245,
0.108859930853323));
#37857=CARTESIAN_POINT('Ctrl Pts',(-0.0968043420335512,0.00361912505495288,
0.109095252915511));
#37858=CARTESIAN_POINT('Ctrl Pts',(-0.0967793169573732,5.66163319584007E-5,
0.109330574977699));
#37859=CARTESIAN_POINT('Origin',(0.,0.,0.1025));
#37860=CARTESIAN_POINT('',(-0.0965227763075221,-6.77612820726425E-6,0.155127758355634));
#37861=CARTESIAN_POINT('',(-0.096524893308144,5.91499715830822E-6,0.149330574977699));
#37862=CARTESIAN_POINT('',(-0.096675,-1.1839272930757E-17,0.1025));
#37863=CARTESIAN_POINT('Ctrl Pts',(-0.0965227763075221,-6.77612820726425E-6,
0.155127758355634));
#37864=CARTESIAN_POINT('Ctrl Pts',(-0.0965190680182828,0.016138816148185,
0.154068559904987));
#37865=CARTESIAN_POINT('Ctrl Pts',(-0.0926787895564408,0.032287429622825,
0.153009361454341));
#37866=CARTESIAN_POINT('Ctrl Pts',(-0.0850136266094788,0.0463495241496994,
0.151950163003694));
#37867=CARTESIAN_POINT('Ctrl Pts',(-0.0698768195982166,0.0741186938986332,
0.14985850720394));
#37868=CARTESIAN_POINT('Ctrl Pts',(-0.0398242971867013,0.0937511675138199,
0.147766851404186));
#37869=CARTESIAN_POINT('Ctrl Pts',(-0.00831514275533874,0.0964661700481194,
0.145675195604432));
#37870=CARTESIAN_POINT('Ctrl Pts',(0.0231940116760242,0.099181172582419,
0.143583539804678));
#37871=CARTESIAN_POINT('Ctrl Pts',(0.0561597981272341,0.0849787040358313,
0.141491884004925));
#37872=CARTESIAN_POINT('Ctrl Pts',(0.0758260807513075,0.0602126271251373,
0.139400228205171));
#37873=CARTESIAN_POINT('Ctrl Pts',(0.0954923633753807,0.0354465502144436,
0.137308572405417));
#37874=CARTESIAN_POINT('Ctrl Pts',(0.101859142172317,0.00011686493964403,
0.135216916605663));
#37875=CARTESIAN_POINT('Ctrl Pts',(0.0920747404299595,-0.0299571361985723,
0.13312526080591));
#37876=CARTESIAN_POINT('Ctrl Pts',(0.0822903386876017,-0.0600311373367887,
0.131033605006156));
#37877=CARTESIAN_POINT('Ctrl Pts',(0.0563547564059492,-0.0848494543384221,
0.128941949206402));
#37878=CARTESIAN_POINT('Ctrl Pts',(0.0258799039839752,-0.0933022984116978,
0.126850293406648));
#37879=CARTESIAN_POINT('Ctrl Pts',(-0.00459494843799892,-0.101755142484973,
0.124758637606895));
#37880=CARTESIAN_POINT('Ctrl Pts',(-0.0396090710002945,-0.0938425136298918,
0.122666981807141));
#37881=CARTESIAN_POINT('Ctrl Pts',(-0.0634871700800987,-0.0731062006114135,
0.120575326007387));
#37882=CARTESIAN_POINT('Ctrl Pts',(-0.0842167694319298,-0.0551041201497079,
0.118759470123469));
#37883=CARTESIAN_POINT('Ctrl Pts',(-0.0965534609291739,-0.0274371894199573,
0.116943614239552));
#37884=CARTESIAN_POINT('Ctrl Pts',(-0.0967646650617208,6.3821447323616E-5,
0.115127758355634));
#37885=CARTESIAN_POINT('Ctrl Pts',(-0.0967793169573732,5.66163319584007E-5,
0.109330574977699));
#37886=CARTESIAN_POINT('Ctrl Pts',(-0.0965819071065392,-0.0280461678752784,
0.111186908715265));
#37887=CARTESIAN_POINT('Ctrl Pts',(-0.0836201771217612,-0.056307862064192,
0.113043242452831));
#37888=CARTESIAN_POINT('Ctrl Pts',(-0.0620812934444443,-0.0743037478312695,
0.114899576190397));
#37889=CARTESIAN_POINT('Ctrl Pts',(-0.0378119877413892,-0.0945809200200219,
0.116991231990151));
#37890=CARTESIAN_POINT('Ctrl Pts',(-0.00265309238045642,-0.101824579550907,
0.119082887789904));
#37891=CARTESIAN_POINT('Ctrl Pts',(0.0276549125922369,-0.0927918697411059,
0.121174543589658));
#37892=CARTESIAN_POINT('Ctrl Pts',(0.0579629175649301,-0.0837591599313047,
0.123266199389412));
#37893=CARTESIAN_POINT('Ctrl Pts',(0.0834200321493839,-0.0584500807808171,
0.125357855189166));
#37894=CARTESIAN_POINT('Ctrl Pts',(0.0926291959676316,-0.0281951895719809,
0.127449510988919));
#37895=CARTESIAN_POINT('Ctrl Pts',(0.101838359785879,0.00205970163685511,
0.129541166788673));
#37896=CARTESIAN_POINT('Ctrl Pts',(0.0947995728379207,0.0372604049040397,
0.131632822588427));
#37897=CARTESIAN_POINT('Ctrl Pts',(0.0746641789865216,0.0616473760057519,
0.133724478388181));
#37898=CARTESIAN_POINT('Ctrl Pts',(0.0545287851351224,0.086034347107464,
0.135816134187934));
#37899=CARTESIAN_POINT('Ctrl Pts',(0.0212967843802825,0.0996075860437037,
0.137907789987688));
#37900=CARTESIAN_POINT('Ctrl Pts',(-0.0101542637302986,0.0962911245681284,
0.139999445787442));
#37901=CARTESIAN_POINT('Ctrl Pts',(-0.04160531184088,0.0929746630925531,
0.142091101587196));
#37902=CARTESIAN_POINT('Ctrl Pts',(-0.0712754073072026,0.0727685012051628,
0.14418275738695));
#37903=CARTESIAN_POINT('Ctrl Pts',(-0.0858809318046248,0.0447174974277489,
0.146274413186703));
#37904=CARTESIAN_POINT('Ctrl Pts',(-0.092994410340263,0.0310555290876898,
0.147293133783702));
#37905=CARTESIAN_POINT('Ctrl Pts',(-0.0965344488013378,0.0155326997615265,
0.148311854380701));
#37906=CARTESIAN_POINT('Ctrl Pts',(-0.096524893308144,5.91499715830822E-6,
0.149330574977699));
#37907=CARTESIAN_POINT('Origin',(0.,0.,-0.0517230892635719));
#37908=CARTESIAN_POINT('',(-0.0737836376428848,-5.17978665142374E-6,0.168276910736428));
#37909=CARTESIAN_POINT('',(-0.0739538094612803,-8.06377484251428E-5,0.176181422596906));
#37910=CARTESIAN_POINT('',(-0.0739,-5.47916578054271E-16,-0.0517230892635719));
#37911=CARTESIAN_POINT('',(0.0526484240822812,-0.0518589764809553,0.183325));
#37912=CARTESIAN_POINT('Ctrl Pts',(-0.0737836376428848,-5.17978665143075E-6,
0.168276910736428));
#37913=CARTESIAN_POINT('Ctrl Pts',(-0.0737864007558564,-0.0120355508218365,
0.169309368085535));
#37914=CARTESIAN_POINT('Ctrl Pts',(-0.0653630139236587,-0.0484316160730116,
0.172433481234396));
#37915=CARTESIAN_POINT('Ctrl Pts',(-0.0107526223003796,-0.085088910335128,
0.177449510988919));
#37916=CARTESIAN_POINT('Ctrl Pts',(0.0372917034486422,-0.0674107586613021,
0.181433083394337));
#37917=CARTESIAN_POINT('Ctrl Pts',(0.0527465304496822,-0.0519092684691894,
0.183325));
#37918=CARTESIAN_POINT('',(-0.0320564751923869,-0.0665852265764703,0.183325));
#37919=CARTESIAN_POINT('Origin',(0.,0.,0.183325));
#37920=CARTESIAN_POINT('Ctrl Pts',(-0.0739538094612803,-8.06377484251584E-5,
0.176181422596905));
#37921=CARTESIAN_POINT('Ctrl Pts',(-0.0739806943658403,-0.00343112332502641,
0.17647095926485));
#37922=CARTESIAN_POINT('Ctrl Pts',(-0.0722722019339485,-0.0309470627246392,
0.178852151732548));
#37923=CARTESIAN_POINT('Ctrl Pts',(-0.0539334858338623,-0.0560528624925751,
0.181233344200246));
#37924=CARTESIAN_POINT('Ctrl Pts',(-0.0320564751923869,-0.0665852265764703,
0.183325));
#37925=CARTESIAN_POINT('Origin',(0.,0.,-0.0517230892635719));
#37926=CARTESIAN_POINT('',(-0.0739685414849875,4.87861904026652E-5,0.128276910736428));
#37927=CARTESIAN_POINT('',(-0.0737852559138541,4.5215235579335E-6,0.136181422596905));
#37928=CARTESIAN_POINT('',(-0.0739,-5.47916578054271E-16,-0.0517230892635719));
#37929=CARTESIAN_POINT('Ctrl Pts',(-0.0739685414849875,4.87861904026683E-5,
0.128276910736428));
#37930=CARTESIAN_POINT('Ctrl Pts',(-0.0738070934850369,-0.0209734502005159,
0.130092766620346));
#37931=CARTESIAN_POINT('Ctrl Pts',(-0.0535140180485454,-0.0664837973240077,
0.134000278304017));
#37932=CARTESIAN_POINT('Ctrl Pts',(0.0232529295866107,-0.0838318934784593,
0.139999445787442));
#37933=CARTESIAN_POINT('Ctrl Pts',(0.0827297187445345,-0.0269172735740158,
0.146274413186704));
#37934=CARTESIAN_POINT('Ctrl Pts',(0.0681290995639721,0.0541025477388684,
0.152549380585964));
#37935=CARTESIAN_POINT('Ctrl Pts',(-0.00746970939628905,0.0866723669969857,
0.158824347985226));
#37936=CARTESIAN_POINT('Ctrl Pts',(-0.0650481952386638,0.0490579501895072,
0.16406685803538));
#37937=CARTESIAN_POINT('Ctrl Pts',(-0.0737808029640662,0.0123367831740457,
0.167217712285781));
#37938=CARTESIAN_POINT('Ctrl Pts',(-0.0737836376428848,-5.17978665143075E-6,
0.168276910736428));
#37939=CARTESIAN_POINT('Ctrl Pts',(-0.0737852559138541,4.52152355793177E-6,
0.136181422596905));
#37940=CARTESIAN_POINT('Ctrl Pts',(-0.0737775628068568,-0.0124960594610031,
0.137254357799661));
#37941=CARTESIAN_POINT('Ctrl Pts',(-0.0648773893377903,-0.049376049988601,
0.140418948802169));
#37942=CARTESIAN_POINT('Ctrl Pts',(-0.00691203799135788,-0.0867186372176302,
0.145675195604432));
#37943=CARTESIAN_POINT('Ctrl Pts',(0.0684817521676531,-0.0536662275708332,
0.151950163003693));
#37944=CARTESIAN_POINT('Ctrl Pts',(0.0825479194741534,0.0274661288420571,
0.158225130402955));
#37945=CARTESIAN_POINT('Ctrl Pts',(0.0227200964169887,0.0839526628083412,
0.164500097802216));
#37946=CARTESIAN_POINT('Ctrl Pts',(-0.0537857498481575,0.0662280371199278,
0.170485528533533));
#37947=CARTESIAN_POINT('Ctrl Pts',(-0.073786473830846,0.0207732810360634,
0.174379303465096));
#37948=CARTESIAN_POINT('Ctrl Pts',(-0.0739538094612803,-8.06377484251584E-5,
0.176181422596905));
#37949=CARTESIAN_POINT('Origin',(0.,0.,-0.0517230892635719));
#37950=CARTESIAN_POINT('',(-0.073893021924492,-6.34491728151829E-5,0.088276910736428));
#37951=CARTESIAN_POINT('',(-0.0739797416410642,4.32784787348095E-5,0.0961814225969055));
#37952=CARTESIAN_POINT('',(-0.0739,-5.47916578054271E-16,-0.0517230892635719));
#37953=CARTESIAN_POINT('Ctrl Pts',(-0.073893021924492,-6.34491728151998E-5,
0.0882769107364281));
#37954=CARTESIAN_POINT('Ctrl Pts',(-0.073944557175508,-0.00595548399039915,
0.0887845093554026));
#37955=CARTESIAN_POINT('Ctrl Pts',(-0.0706303381894479,-0.0360694472427554,
0.0913837637741309));
#37956=CARTESIAN_POINT('Ctrl Pts',(-0.0294984946271671,-0.081844073714394,
0.0960746739926129));
#37957=CARTESIAN_POINT('Ctrl Pts',(0.0519368418851493,-0.0697937884462804,
0.102349641391874));
#37958=CARTESIAN_POINT('Ctrl Pts',(0.0868678567944775,0.00474910384924522,
0.108624608791136));
#37959=CARTESIAN_POINT('Ctrl Pts',(0.0440185536514787,0.0750397778351934,
0.114899576190397));
#37960=CARTESIAN_POINT('Ctrl Pts',(-0.0382446064732518,0.078140441559687,
0.121174543589658));
#37961=CARTESIAN_POINT('Ctrl Pts',(-0.0723681031162574,0.0306247471374611,
0.125633655105002));
#37962=CARTESIAN_POINT('Ctrl Pts',(-0.0739930628939785,0.00324173287667585,
0.128001110820592));
#37963=CARTESIAN_POINT('Ctrl Pts',(-0.0739685414849875,4.87861904026683E-5,
0.128276910736428));
#37964=CARTESIAN_POINT('Ctrl Pts',(-0.0739797416410642,4.32784787348099E-5,
0.0961814225969055));
#37965=CARTESIAN_POINT('Ctrl Pts',(-0.073828838222635,-0.0214389635995149,
0.0980377563344713));
#37966=CARTESIAN_POINT('Ctrl Pts',(-0.0527564789060794,-0.0673850352691751,
0.101985745871791));
#37967=CARTESIAN_POINT('Ctrl Pts',(0.0248479838661208,-0.0833736009117604,
0.108025391208864));
#37968=CARTESIAN_POINT('Ctrl Pts',(0.0832275266990493,-0.0253335404239085,
0.114300358608126));
#37969=CARTESIAN_POINT('Ctrl Pts',(0.0670858244351509,0.0553904928249651,
0.120575326007387));
#37970=CARTESIAN_POINT('Ctrl Pts',(-0.00912348063180574,0.0865173309130365,
0.126850293406648));
#37971=CARTESIAN_POINT('Ctrl Pts',(-0.0655303527769235,0.0481026789811179,
0.132052325603154));
#37972=CARTESIAN_POINT('Ctrl Pts',(-0.0737925602939629,0.0118734575885883,
0.135162701999907));
#37973=CARTESIAN_POINT('Ctrl Pts',(-0.0737852559138541,4.52152355793177E-6,
0.136181422596905));
#37974=CARTESIAN_POINT('Origin',(0.,0.,-0.0517230892635719));
#37975=CARTESIAN_POINT('',(-0.0738258018559393,4.09328341953636E-5,0.0482769107364281));
#37976=CARTESIAN_POINT('',(-0.0738797477720541,-6.29004154842697E-5,0.0561814225969054));
#37977=CARTESIAN_POINT('',(-0.0739,-5.47916578054271E-16,-0.0517230892635719));
#37978=CARTESIAN_POINT('Ctrl Pts',(-0.0738258018559393,4.09328341953522E-5,
0.0482769107364281));
#37979=CARTESIAN_POINT('Ctrl Pts',(-0.0737420584453234,-0.0149871305718488,
0.0495679078902133));
#37980=CARTESIAN_POINT('Ctrl Pts',(-0.0619974316400658,-0.054474758919102,
0.0529505608437523));
#37981=CARTESIAN_POINT('Ctrl Pts',(0.00200588979265343,-0.0869742751577483,
0.0584248695970452));
#37982=CARTESIAN_POINT('Ctrl Pts',(0.0736302858054235,-0.0463507894749077,
0.0646998369963064));
#37983=CARTESIAN_POINT('Ctrl Pts',(0.079297411853797,0.0357745193205231,
0.0709748043955678));
#37984=CARTESIAN_POINT('Ctrl Pts',(0.0139779125109316,0.0858677928042342,
0.077249771794829));
#37985=CARTESIAN_POINT('Ctrl Pts',(-0.0575684509810804,0.0612431240737476,
0.0830171405751159));
#37986=CARTESIAN_POINT('Ctrl Pts',(-0.0737321964584969,0.0183237562160622,
0.0866928535556488));
#37987=CARTESIAN_POINT('Ctrl Pts',(-0.073893021924492,-6.34491728151998E-5,
0.0882769107364281));
#37988=CARTESIAN_POINT('Ctrl Pts',(-0.0738797477720541,-6.29004154842593E-5,
0.0561814225969054));
#37989=CARTESIAN_POINT('Ctrl Pts',(-0.0739335770439367,-0.00642783008921347,
0.0567294990695283));
#37990=CARTESIAN_POINT('Ctrl Pts',(-0.0702896161667766,-0.0370223588314532,
0.0593692313419049));
#37991=CARTESIAN_POINT('Ctrl Pts',(-0.027934008198508,-0.0823914539723853,
0.0641006194140353));
#37992=CARTESIAN_POINT('Ctrl Pts',(0.0532596375466719,-0.0687906809299483,
0.0703755868132967));
#37993=CARTESIAN_POINT('Ctrl Pts',(0.0867609319023758,0.00640524336665911,
0.0766505542125579));
#37994=CARTESIAN_POINT('Ctrl Pts',(0.0425795741016805,0.0758656338855472,
0.0829255216118193));
#37995=CARTESIAN_POINT('Ctrl Pts',(-0.0397282592051405,0.0773968661599418,
0.0892004890110804));
#37996=CARTESIAN_POINT('Ctrl Pts',(-0.0726375375548605,0.0296759427852165,
0.093619122672776));
#37997=CARTESIAN_POINT('Ctrl Pts',(-0.0739988712312329,0.00276652021268154,
0.0959461005347176));
#37998=CARTESIAN_POINT('Ctrl Pts',(-0.0739797416410642,4.32784787348099E-5,
0.0961814225969055));
#37999=CARTESIAN_POINT('Origin',(2.39206768658147E-17,-5.43753587379397E-18,
0.183325));
#38000=CARTESIAN_POINT('',(0.0270116869336341,0.092824697112349,0.183325));
#38001=CARTESIAN_POINT('Ctrl Pts',(0.0527465304496837,-0.0519092684691879,
0.183325));
#38002=CARTESIAN_POINT('Ctrl Pts',(0.0546401156765816,-0.0505045722914166,
0.183325));
#38003=CARTESIAN_POINT('Ctrl Pts',(0.0564577449202127,-0.0490079002578489,
0.183325));
#38004=CARTESIAN_POINT('Ctrl Pts',(0.0581912954394417,-0.0474228118599484,
0.183325));
#38005=CARTESIAN_POINT('Ctrl Pts',(0.0613530156193595,-0.0445318629553705,
0.183325));
#38006=CARTESIAN_POINT('Ctrl Pts',(0.0642355283205663,-0.0413475100044657,
0.183325));
#38007=CARTESIAN_POINT('Ctrl Pts',(0.066834120121686,-0.0379215868621348,
0.183325));
#38008=CARTESIAN_POINT('Ctrl Pts',(0.0685601271369542,-0.0356460592571895,
0.183325));
#38009=CARTESIAN_POINT('Ctrl Pts',(0.0701548344174317,-0.0332713934661594,
0.183325));
#38010=CARTESIAN_POINT('Ctrl Pts',(0.0716166500276835,-0.0308145965037307,
0.183325));
#38011=CARTESIAN_POINT('Ctrl Pts',(0.0732633814775101,-0.0280470211710436,
0.183325));
#38012=CARTESIAN_POINT('Ctrl Pts',(0.0747419256656459,-0.0251747141098478,
0.183325));
#38013=CARTESIAN_POINT('Ctrl Pts',(0.0760495595769769,-0.0222174250112788,
0.183325));
#38014=CARTESIAN_POINT('Ctrl Pts',(0.0771636755795777,-0.0196977877638178,
0.183325));
#38015=CARTESIAN_POINT('Ctrl Pts',(0.0781534655055068,-0.0171156032244178,
0.183325));
#38016=CARTESIAN_POINT('Ctrl Pts',(0.0790121194120802,-0.0144979013638344,
0.183325));
#38017=CARTESIAN_POINT('Ctrl Pts',(0.0811176435774726,-0.00807897694847167,
0.183325));
#38018=CARTESIAN_POINT('Ctrl Pts',(0.0824473371994335,-0.00142879370438768,
0.183325));
#38019=CARTESIAN_POINT('Ctrl Pts',(0.0829720082147319,0.00528756526002575,
0.183325));
#38020=CARTESIAN_POINT('Ctrl Pts',(0.0831605422866328,0.00770100619155721,
0.183325));
#38021=CARTESIAN_POINT('Ctrl Pts',(0.0832446865927584,0.0101257041339963,
0.183325));
#38022=CARTESIAN_POINT('Ctrl Pts',(0.0832217255425897,0.0125466916461908,
0.183325));
#38023=CARTESIAN_POINT('Ctrl Pts',(0.0831801213734689,0.0169333888206161,
0.183325));
#38024=CARTESIAN_POINT('Ctrl Pts',(0.082788129105151,0.0212914783977859,
0.183325));
#38025=CARTESIAN_POINT('Ctrl Pts',(0.0820392315336429,0.0255780886223147,
0.183325));
#38026=CARTESIAN_POINT('Ctrl Pts',(0.0811462944344166,0.0306891658176867,
0.183325));
#38027=CARTESIAN_POINT('Ctrl Pts',(0.0797466521321354,0.0356990115058088,
0.183325));
#38028=CARTESIAN_POINT('Ctrl Pts',(0.077891263133679,0.0405655957602974,
0.183325));
#38029=CARTESIAN_POINT('Ctrl Pts',(0.0769495055492577,0.0430357745937942,
0.183325));
#38030=CARTESIAN_POINT('Ctrl Pts',(0.0758888412672695,0.0454706621806907,
0.183325));
#38031=CARTESIAN_POINT('Ctrl Pts',(0.0747230976172314,0.0478488836962904,
0.183325));
#38032=CARTESIAN_POINT('Ctrl Pts',(0.0722755117057051,0.0528421782991648,
0.183325));
#38033=CARTESIAN_POINT('Ctrl Pts',(0.0693611729291524,0.0576008143227626,
0.183325));
#38034=CARTESIAN_POINT('Ctrl Pts',(0.0660414991224629,0.0620762069120578,
0.183325));
#38035=CARTESIAN_POINT('Ctrl Pts',(0.0634288730603047,0.0655983985483629,
0.183325));
#38036=CARTESIAN_POINT('Ctrl Pts',(0.0605647053893801,0.0689452797930669,
0.183325));
#38037=CARTESIAN_POINT('Ctrl Pts',(0.0574711285697693,0.0720908849414506,
0.183325));
#38038=CARTESIAN_POINT('Ctrl Pts',(0.0555574201065491,0.0740367784962025,
0.183325));
#38039=CARTESIAN_POINT('Ctrl Pts',(0.0535622771425319,0.0758988193647838,
0.183325));
#38040=CARTESIAN_POINT('Ctrl Pts',(0.0514951532726063,0.0776691885827886,
0.183325));
#38041=CARTESIAN_POINT('Ctrl Pts',(0.0457945092115925,0.0825514527350495,
0.183325));
#38042=CARTESIAN_POINT('Ctrl Pts',(0.0395430238483871,0.0867452732609154,
0.183325));
#38043=CARTESIAN_POINT('Ctrl Pts',(0.0328518740906454,0.0901282422580833,
0.183325));
#38044=CARTESIAN_POINT('Ctrl Pts',(0.0309405875159093,0.0910945669498233,
0.183325));
#38045=CARTESIAN_POINT('Ctrl Pts',(0.028993174707338,0.0919945319583493,
0.183325));
#38046=CARTESIAN_POINT('Ctrl Pts',(0.0270116869336341,0.0928246971123491,
0.183325));
#38047=CARTESIAN_POINT('',(-0.096675,-1.1839272930757E-17,0.183325));
#38048=CARTESIAN_POINT('Origin',(0.,0.,0.183325));
#38049=CARTESIAN_POINT('',(-0.0568713879600425,0.0783474662532323,0.183325));
#38050=CARTESIAN_POINT('Origin',(0.,0.,0.183325));
#38051=CARTESIAN_POINT('Ctrl Pts',(-0.0568713879600414,0.0783474662532331,
0.183325));
#38052=CARTESIAN_POINT('Ctrl Pts',(-0.0591169345770589,0.076315216152872,
0.183325));
#38053=CARTESIAN_POINT('Ctrl Pts',(-0.0612562739924736,0.0741756319431535,
0.183325));
#38054=CARTESIAN_POINT('Ctrl Pts',(-0.0632787201244711,0.0719302794170955,
0.183325));
#38055=CARTESIAN_POINT('Ctrl Pts',(-0.0669251707984549,0.0678819306861015,
0.183325));
#38056=CARTESIAN_POINT('Ctrl Pts',(-0.0701924279121554,0.0634898239153897,
0.183325));
#38057=CARTESIAN_POINT('Ctrl Pts',(-0.0730590010288785,0.0588183271803977,
0.183325));
#38058=CARTESIAN_POINT('Ctrl Pts',(-0.0746566708643339,0.0562146924165105,
0.183325));
#38059=CARTESIAN_POINT('Ctrl Pts',(-0.0761246913269906,0.0535322363953255,
0.183325));
#38060=CARTESIAN_POINT('Ctrl Pts',(-0.0774597304405968,0.0507837216288562,
0.183325));
#38061=CARTESIAN_POINT('Ctrl Pts',(-0.0796092977453778,0.0463582951237468,
0.183325));
#38062=CARTESIAN_POINT('Ctrl Pts',(-0.0814151665646452,0.0417606422657594,
0.183325));
#38063=CARTESIAN_POINT('Ctrl Pts',(-0.0828578508387229,0.0370391959667551,
0.183325));
#38064=CARTESIAN_POINT('Ctrl Pts',(-0.0836414140099655,0.0344748431825919,
0.183325));
#38065=CARTESIAN_POINT('Ctrl Pts',(-0.0843160631417445,0.0318785210818391,
0.183325));
#38066=CARTESIAN_POINT('Ctrl Pts',(-0.0848776834159108,0.0292657100558518,
0.183325));
#38067=CARTESIAN_POINT('Ctrl Pts',(-0.0863774880178461,0.0222882090983227,
0.183325));
#38068=CARTESIAN_POINT('Ctrl Pts',(-0.0870800845145338,0.01517559244937,
0.183325));
#38069=CARTESIAN_POINT('Ctrl Pts',(-0.08691711176372,0.00808290042294868,
0.183325));
#38070=CARTESIAN_POINT('Ctrl Pts',(-0.086829761851914,0.00428136906337395,
0.183325));
#38071=CARTESIAN_POINT('Ctrl Pts',(-0.0864910968448572,0.000479251015311818,
0.183325));
#38072=CARTESIAN_POINT('Ctrl Pts',(-0.0858921759183976,-0.00326140466639689,
0.183325));
#38073=CARTESIAN_POINT('Ctrl Pts',(-0.0854431276238688,-0.00606600704390875,
0.183325));
#38074=CARTESIAN_POINT('Ctrl Pts',(-0.084848151198669,-0.00883918603235441,
0.183325));
#38075=CARTESIAN_POINT('Ctrl Pts',(-0.0841024998475747,-0.0115704941964249,
0.183325));
#38076=CARTESIAN_POINT('Ctrl Pts',(-0.08282572696136,-0.0162472914726108,
0.183325));
#38077=CARTESIAN_POINT('Ctrl Pts',(-0.0811075596191732,-0.0208019296013592,
0.183325));
#38078=CARTESIAN_POINT('Ctrl Pts',(-0.0789832762820567,-0.0251872000190629,
0.183325));
#38079=CARTESIAN_POINT('Ctrl Pts',(-0.0776463058116779,-0.0279471788555274,
0.183325));
#38080=CARTESIAN_POINT('Ctrl Pts',(-0.0761461905929749,-0.0306420990887643,
0.183325));
#38081=CARTESIAN_POINT('Ctrl Pts',(-0.0745048321361633,-0.0332382132025085,
0.183325));
#38082=CARTESIAN_POINT('Ctrl Pts',(-0.0720489128888603,-0.037122706923962,
0.183325));
#38083=CARTESIAN_POINT('Ctrl Pts',(-0.0692726962881112,-0.0407973756999029,
0.183325));
#38084=CARTESIAN_POINT('Ctrl Pts',(-0.0662082873966704,-0.0442215373549909,
0.183325));
#38085=CARTESIAN_POINT('Ctrl Pts',(-0.0638653650588976,-0.0468395120163549,
0.183325));
#38086=CARTESIAN_POINT('Ctrl Pts',(-0.0613537638211011,-0.0493109066276996,
0.183325));
#38087=CARTESIAN_POINT('Ctrl Pts',(-0.0586860692431017,-0.0516129350947554,
0.183325));
#38088=CARTESIAN_POINT('Ctrl Pts',(-0.0569207005495688,-0.0531363212503061,
0.183325));
#38089=CARTESIAN_POINT('Ctrl Pts',(-0.0550890271379007,-0.0545832784834442,
0.183325));
#38090=CARTESIAN_POINT('Ctrl Pts',(-0.0532033891510083,-0.0559417504951859,
0.183325));
#38091=CARTESIAN_POINT('Ctrl Pts',(-0.0482461350711257,-0.0595131098809348,
0.183325));
#38092=CARTESIAN_POINT('Ctrl Pts',(-0.0429006042715654,-0.0624903801211849,
0.183325));
#38093=CARTESIAN_POINT('Ctrl Pts',(-0.0372392688433482,-0.0647497023123468,
0.183325));
#38094=CARTESIAN_POINT('Ctrl Pts',(-0.0355395009110826,-0.0654280446324383,
0.183325));
#38095=CARTESIAN_POINT('Ctrl Pts',(-0.0338112391786412,-0.0660413200514086,
0.183325));
#38096=CARTESIAN_POINT('Ctrl Pts',(-0.0320564751923869,-0.0665852265764703,
0.183325));
#38097=CARTESIAN_POINT('Ctrl Pts',(-0.0598243716961198,-0.0433849576600519,
0.0201758476192062));
#38098=CARTESIAN_POINT('Ctrl Pts',(-0.0455699607823283,-0.0630406453179218,
0.02226750341896));
#38099=CARTESIAN_POINT('Ctrl Pts',(0.00356195933852505,-0.0869026068573454,
0.0264508150184675));
#38100=CARTESIAN_POINT('Ctrl Pts',(0.0745504773406983,-0.0449472636719899,
0.0327257824177288));
#38101=CARTESIAN_POINT('Ctrl Pts',(0.0785751349489661,0.0372853931394063,
0.0390007498169901));
#38102=CARTESIAN_POINT('Ctrl Pts',(0.0123509105275246,0.0861162136430816,
0.0452757172162514));
#38103=CARTESIAN_POINT('Ctrl Pts',(-0.0649875833194373,0.0578483221531574,
0.0515506846155127));
#38104=CARTESIAN_POINT('Ctrl Pts',(-0.0841078107116264,-0.022221037045425,
0.057825652014774));
#38105=CARTESIAN_POINT('Ctrl Pts',(-0.027934008198508,-0.0823914539723853,
0.0641006194140353));
#38106=CARTESIAN_POINT('Ctrl Pts',(0.0532596375466719,-0.0687906809299483,
0.0703755868132967));
#38107=CARTESIAN_POINT('Ctrl Pts',(0.0867609319023758,0.00640524336665911,
0.0766505542125579));
#38108=CARTESIAN_POINT('Ctrl Pts',(0.0425795741016805,0.0758656338855472,
0.0829255216118193));
#38109=CARTESIAN_POINT('Ctrl Pts',(-0.0397282592051405,0.0773968661599418,
0.0892004890110804));
#38110=CARTESIAN_POINT('Ctrl Pts',(-0.0864632149829576,0.00962767292835096,
0.0954754564103419));
#38111=CARTESIAN_POINT('Ctrl Pts',(-0.0557801733774148,-0.0667620744778611,
0.101750423809603));
#38112=CARTESIAN_POINT('Ctrl Pts',(0.0248479838661208,-0.0833736009117604,
0.108025391208864));
#38113=CARTESIAN_POINT('Ctrl Pts',(0.0832275266990493,-0.0253335404239085,
0.114300358608126));
#38114=CARTESIAN_POINT('Ctrl Pts',(0.0670858244351509,0.0553904928249651,
0.120575326007387));
#38115=CARTESIAN_POINT('Ctrl Pts',(-0.00912348063180574,0.0865173309130365,
0.126850293406648));
#38116=CARTESIAN_POINT('Ctrl Pts',(-0.0771644443233876,0.0401795384078964,
0.13312526080591));
#38117=CARTESIAN_POINT('Ctrl Pts',(-0.0761117357355759,-0.0421386305548231,
0.139400228205171));
#38118=CARTESIAN_POINT('Ctrl Pts',(-0.00691203799135788,-0.0867186372176302,
0.145675195604432));
#38119=CARTESIAN_POINT('Ctrl Pts',(0.0684817521676531,-0.0536662275708332,
0.151950163003693));
#38120=CARTESIAN_POINT('Ctrl Pts',(0.0825479194741534,0.0274661288420571,
0.158225130402955));
#38121=CARTESIAN_POINT('Ctrl Pts',(0.0227200964169887,0.0839526628083412,
0.164500097802216));
#38122=CARTESIAN_POINT('Ctrl Pts',(-0.0574866109557766,0.065370633652616,
0.170775065201478));
#38123=CARTESIAN_POINT('Ctrl Pts',(-0.0861511939033514,-0.0119466489844985,
0.177050032600739));
#38124=CARTESIAN_POINT('Ctrl Pts',(-0.0539334858338623,-0.0560528624925751,
0.181233344200246));
#38125=CARTESIAN_POINT('Ctrl Pts',(-0.0320564751923869,-0.0665852265764703,
0.183325));
#38126=CARTESIAN_POINT('Ctrl Pts',(-0.0659700643681051,-0.0478418471986522,
0.0245588984128041));
#38127=CARTESIAN_POINT('Ctrl Pts',(-0.0502513133164625,-0.0695167422828098,
0.0266505542125579));
#38128=CARTESIAN_POINT('Ctrl Pts',(0.00392787554932748,-0.0958300171919238,
0.0308338658120655));
#38129=CARTESIAN_POINT('Ctrl Pts',(0.0822089668374704,-0.0495646472088848,
0.0371088332113267));
#38130=CARTESIAN_POINT('Ctrl Pts',(0.0866470731468132,0.0411156810453602,
0.043383800610588));
#38131=CARTESIAN_POINT('Ctrl Pts',(0.0136197061399035,0.094962838657611,
0.0496587680098493));
#38132=CARTESIAN_POINT('Ctrl Pts',(-0.0716636871087931,0.063791017403668,
0.0559337354091106));
#38133=CARTESIAN_POINT('Ctrl Pts',(-0.0927481146762511,-0.0245037800256215,
0.062208702808372));
#38134=CARTESIAN_POINT('Ctrl Pts',(-0.0308036384949493,-0.0908554384749611,
0.0684836702076331));
#38135=CARTESIAN_POINT('Ctrl Pts',(0.0587309422157087,-0.0758574728026573,
0.0747586376068946));
#38136=CARTESIAN_POINT('Ctrl Pts',(0.0956737881228386,0.00706324705486688,
0.0810336050061558));
#38137=CARTESIAN_POINT('Ctrl Pts',(0.0469537274628253,0.0836592279845247,
0.0873085724054171));
#38138=CARTESIAN_POINT('Ctrl Pts',(-0.0438095000864985,0.0853477620859351,
0.0935835398046784));
#38139=CARTESIAN_POINT('Ctrl Pts',(-0.0953454870679233,0.0106167133024745,
0.0998585072039397));
#38140=CARTESIAN_POINT('Ctrl Pts',(-0.0615104099523837,-0.073620469814953,
0.106133474603201));
#38141=CARTESIAN_POINT('Ctrl Pts',(0.0274005902375725,-0.091938480301771,
0.112408442002462));
#38142=CARTESIAN_POINT('Ctrl Pts',(0.0917774000439788,-0.0279360274927155,
0.118683409401724));
#38143=CARTESIAN_POINT('Ctrl Pts',(0.0739774782534214,0.0610806979403848,
0.124958376800985));
#38144=CARTESIAN_POINT('Ctrl Pts',(-0.0100607258793897,0.0954051622686722,
0.131233344200246));
#38145=CARTESIAN_POINT('Ctrl Pts',(-0.0850914638067668,0.0443071387111884,
0.137508311599508));
#38146=CARTESIAN_POINT('Ctrl Pts',(-0.0839306116100808,-0.0464674862647287,
0.143783278998769));
#38147=CARTESIAN_POINT('Ctrl Pts',(-0.00762210414044755,-0.0956271485511058,
0.15005824639803));
#38148=CARTESIAN_POINT('Ctrl Pts',(0.0755168081244337,-0.0591793007910665,
0.156333213797291));
#38149=CARTESIAN_POINT('Ctrl Pts',(0.0910279775076395,0.0302876944008205,
0.162608181196553));
#38150=CARTESIAN_POINT('Ctrl Pts',(0.0250541072239211,0.0925770285975157,
0.168883148595814));
#38151=CARTESIAN_POINT('Ctrl Pts',(-0.0633921480081798,0.0720860877863026,
0.175158115995075));
#38152=CARTESIAN_POINT('Ctrl Pts',(-0.0950014124019929,-0.0131739152480164,
0.181433083394337));
#38153=CARTESIAN_POINT('Ctrl Pts',(-0.0594740142049323,-0.0618111121239165,
0.185616394993844));
#38154=CARTESIAN_POINT('Ctrl Pts',(-0.0353496020417627,-0.0734254545208957,
0.187708050793598));
#38155=CARTESIAN_POINT('Ctrl Pts',(-0.0721157570400904,-0.0522987367372524,
0.028941949206402));
#38156=CARTESIAN_POINT('Ctrl Pts',(-0.0549326658505966,-0.0759928392476978,
0.0310336050061558));
#38157=CARTESIAN_POINT('Ctrl Pts',(0.00429379176012989,-0.104757427526502,
0.0352169166056634));
#38158=CARTESIAN_POINT('Ctrl Pts',(0.0898674563342426,-0.0541820307457796,
0.0414918840049246));
#38159=CARTESIAN_POINT('Ctrl Pts',(0.0947190113446605,0.044945968951314,
0.047766851404186));
#38160=CARTESIAN_POINT('Ctrl Pts',(0.0148885017522822,0.103809463672141,
0.0540418188034472));
#38161=CARTESIAN_POINT('Ctrl Pts',(-0.0783397908981488,0.0697337126541784,
0.0603167862027086));
#38162=CARTESIAN_POINT('Ctrl Pts',(-0.101388418640876,-0.0267865230058178,
0.0665917536019698));
#38163=CARTESIAN_POINT('Ctrl Pts',(-0.0336732687913905,-0.099319422977537,
0.0728667210012312));
#38164=CARTESIAN_POINT('Ctrl Pts',(0.0642022468847453,-0.0829242646753663,
0.0791416884004924));
#38165=CARTESIAN_POINT('Ctrl Pts',(0.104586644343302,0.00772125074307456,
0.0854166557997538));
#38166=CARTESIAN_POINT('Ctrl Pts',(0.0513278808239699,0.0914528220835024,
0.0916916231990151));
#38167=CARTESIAN_POINT('Ctrl Pts',(-0.0478907409678564,0.0932986580119281,
0.0979665905982763));
#38168=CARTESIAN_POINT('Ctrl Pts',(-0.104227759152889,0.0116057536765983,
0.104241557997538));
#38169=CARTESIAN_POINT('Ctrl Pts',(-0.0672406465273527,-0.080478865152045,
0.110516525396799));
#38170=CARTESIAN_POINT('Ctrl Pts',(0.0299531966090245,-0.100503359691781,
0.11679149279606));
#38171=CARTESIAN_POINT('Ctrl Pts',(0.100327273388908,-0.0305385145615227,
0.123066460195322));
#38172=CARTESIAN_POINT('Ctrl Pts',(0.0808691320716919,0.0667709030558047,
0.129341427594583));
#38173=CARTESIAN_POINT('Ctrl Pts',(-0.0109979711269736,0.104292993624308,
0.135616394993844));
#38174=CARTESIAN_POINT('Ctrl Pts',(-0.0930184832901458,0.0484347390144806,
0.141891362393105));
#38175=CARTESIAN_POINT('Ctrl Pts',(-0.0917494874845858,-0.0507963419746343,
0.148166329792367));
#38176=CARTESIAN_POINT('Ctrl Pts',(-0.00833217028953726,-0.104535659884581,
0.154441297191628));
#38177=CARTESIAN_POINT('Ctrl Pts',(0.0825518640812145,-0.0646923740112998,
0.160716264590889));
#38178=CARTESIAN_POINT('Ctrl Pts',(0.0995080355411255,0.0331092599595838,
0.166991231990151));
#38179=CARTESIAN_POINT('Ctrl Pts',(0.0273881180308536,0.10120139438669,
0.173266199389412));
#38180=CARTESIAN_POINT('Ctrl Pts',(-0.0692976850605831,0.0788015419199893,
0.179541166788673));
#38181=CARTESIAN_POINT('Ctrl Pts',(-0.103851630900634,-0.0144011815115344,
0.185816134187935));
#38182=CARTESIAN_POINT('Ctrl Pts',(-0.0650145425760024,-0.0675693617552579,
0.189999445787442));
#38183=CARTESIAN_POINT('Ctrl Pts',(-0.0386427288911385,-0.0802656824653211,
0.192091101587196));
#38184=CARTESIAN_POINT('Ctrl Pts',(-0.0782614497120757,-0.0567556262758526,
0.033325));
#38185=CARTESIAN_POINT('Ctrl Pts',(-0.0596140183847307,-0.0824689362125857,
0.0354166557997537));
#38186=CARTESIAN_POINT('Ctrl Pts',(0.00465970797093226,-0.113684837861081,
0.0395999673992613));
#38187=CARTESIAN_POINT('Ctrl Pts',(0.0975259458310149,-0.0587994142826744,
0.0458749347985225));
#38188=CARTESIAN_POINT('Ctrl Pts',(0.102790949542507,0.0487762568572679,
0.0521499021977838));
#38189=CARTESIAN_POINT('Ctrl Pts',(0.0161572973646611,0.11265608868667,
0.0584248695970452));
#38190=CARTESIAN_POINT('Ctrl Pts',(-0.0850158946875046,0.0756764079046889,
0.0646998369963064));
#38191=CARTESIAN_POINT('Ctrl Pts',(-0.110028722605501,-0.0290692659860142,
0.0709748043955679));
#38192=CARTESIAN_POINT('Ctrl Pts',(-0.0365428990878319,-0.107783407480113,
0.0772497717948288));
#38193=CARTESIAN_POINT('Ctrl Pts',(0.0696735515537822,-0.0899910565480753,
0.0835247391940905));
#38194=CARTESIAN_POINT('Ctrl Pts',(0.113499500563764,0.00837925443128228,
0.0897997065933516));
#38195=CARTESIAN_POINT('Ctrl Pts',(0.0557020341851148,0.0992464161824799,
0.096074673992613));
#38196=CARTESIAN_POINT('Ctrl Pts',(-0.0519719818492145,0.101249553937921,
0.102349641391874));
#38197=CARTESIAN_POINT('Ctrl Pts',(-0.113110031237854,0.0125947940507219,
0.108624608791136));
#38198=CARTESIAN_POINT('Ctrl Pts',(-0.0729708831023218,-0.0873372604891369,
0.114899576190397));
#38199=CARTESIAN_POINT('Ctrl Pts',(0.0325058029804763,-0.109068239081792,
0.121174543589658));
#38200=CARTESIAN_POINT('Ctrl Pts',(0.108877146733838,-0.0331410016303297,
0.127449510988919));
#38201=CARTESIAN_POINT('Ctrl Pts',(0.0877607858899622,0.0724611081712244,
0.133724478388181));
#38202=CARTESIAN_POINT('Ctrl Pts',(-0.0119352163745575,0.113180824979943,
0.139999445787442));
#38203=CARTESIAN_POINT('Ctrl Pts',(-0.100945502773525,0.0525623393177726,
0.146274413186703));
#38204=CARTESIAN_POINT('Ctrl Pts',(-0.0995683633590906,-0.05512519768454,
0.152549380585965));
#38205=CARTESIAN_POINT('Ctrl Pts',(-0.00904223643862709,-0.113444171218057,
0.158824347985226));
#38206=CARTESIAN_POINT('Ctrl Pts',(0.0895869200379953,-0.0702054472315332,
0.165099315384487));
#38207=CARTESIAN_POINT('Ctrl Pts',(0.107988093574611,0.0359308255183472,
0.171374282783748));
#38208=CARTESIAN_POINT('Ctrl Pts',(0.0297221288377862,0.109825760175864,
0.17764925018301));
#38209=CARTESIAN_POINT('Ctrl Pts',(-0.0752032221129864,0.0855169960536761,
0.183924217582271));
#38210=CARTESIAN_POINT('Ctrl Pts',(-0.112701849399276,-0.0156284477750525,
0.190199184981533));
#38211=CARTESIAN_POINT('Ctrl Pts',(-0.0705550709470724,-0.0733276113865993,
0.19438249658104));
#38212=CARTESIAN_POINT('Ctrl Pts',(-0.0419358557405144,-0.0871059104097464,
0.196474152380794));
#38213=CARTESIAN_POINT('Ctrl Pts',(-0.096524893308144,5.91499715830822E-6,
0.149330574977699));
#38214=CARTESIAN_POINT('Ctrl Pts',(-0.0965148292875898,-0.0163471792745932,
0.150403510180454));
#38215=CARTESIAN_POINT('Ctrl Pts',(-0.0925673112842537,-0.0327046611907102,
0.151476445383209));
#38216=CARTESIAN_POINT('Ctrl Pts',(-0.0847101987747527,-0.0468971037730737,
0.152549380585965));
#38217=CARTESIAN_POINT('Ctrl Pts',(-0.0693929877189364,-0.0745648555290454,
0.154641036385718));
#38218=CARTESIAN_POINT('Ctrl Pts',(-0.0392176120787817,-0.0940045133735512,
0.156732692185472));
#38219=CARTESIAN_POINT('Ctrl Pts',(-0.00769173151260052,-0.0965178882980501,
0.158824347985226));
#38220=CARTESIAN_POINT('Ctrl Pts',(0.0238341490535804,-0.0990312632225489,
0.16091600378498));
#38221=CARTESIAN_POINT('Ctrl Pts',(0.0567105345457878,-0.0846183552270411,
0.163007659584734));
#38222=CARTESIAN_POINT('Ctrl Pts',(0.0762155895479942,-0.0597225224376405,
0.165099315384487));
#38223=CARTESIAN_POINT('Ctrl Pts',(0.0957206445502008,-0.0348266896482397,
0.167190971184241));
#38224=CARTESIAN_POINT('Ctrl Pts',(0.101854369062406,0.000552067935053632,
0.169282626983995));
#38225=CARTESIAN_POINT('Ctrl Pts',(0.0918769038623711,0.0305572691696201,
0.171374282783748));
#38226=CARTESIAN_POINT('Ctrl Pts',(0.0818994386623363,0.0605624704041863,
0.173465938583502));
#38227=CARTESIAN_POINT('Ctrl Pts',(0.055810783750061,0.0851941152900256,
0.175557594383256));
#38228=CARTESIAN_POINT('Ctrl Pts',(0.025278897802128,0.0934584770459136,
0.17764925018301));
#38229=CARTESIAN_POINT('Ctrl Pts',(-0.00233739644375865,0.100933647311985,
0.179541166788673));
#38230=CARTESIAN_POINT('Ctrl Pts',(-0.0335888415240724,0.0950182145574911,
0.181433083394336));
#38231=CARTESIAN_POINT('Ctrl Pts',(-0.0568713879600425,0.0783474662532323,
0.183325));
#38232=CARTESIAN_POINT('',(0.0666656654670482,-0.0321318641035092,0.033325));
#38233=CARTESIAN_POINT('Ctrl Pts',(0.0666656654670482,-0.0321318641035094,
0.033325));
#38234=CARTESIAN_POINT('Ctrl Pts',(0.0659824885931634,-0.0343884334763996,
0.033325));
#38235=CARTESIAN_POINT('Ctrl Pts',(0.0651870973984133,-0.0366045459221621,
0.033325));
#38236=CARTESIAN_POINT('Ctrl Pts',(0.0642801010966116,-0.0387713539337305,
0.033325));
#38237=CARTESIAN_POINT('Ctrl Pts',(0.0626258865399732,-0.0427232612866675,
0.033325));
#38238=CARTESIAN_POINT('Ctrl Pts',(0.0606012519142644,-0.0465113694703073,
0.033325));
#38239=CARTESIAN_POINT('Ctrl Pts',(0.0582533982229137,-0.0501137477423414,
0.033325));
#38240=CARTESIAN_POINT('Ctrl Pts',(0.0566939280556225,-0.0525064868926687,
0.033325));
#38241=CARTESIAN_POINT('Ctrl Pts',(0.0549968220046632,-0.0548090897547331,
0.033325));
#38242=CARTESIAN_POINT('Ctrl Pts',(0.053177551929251,-0.0570143177582109,
0.033325));
#38243=CARTESIAN_POINT('Ctrl Pts',(0.0511281594918407,-0.0594984885551547,
0.033325));
#38244=CARTESIAN_POINT('Ctrl Pts',(0.048923417608628,-0.0618596889026584,
0.033325));
#38245=CARTESIAN_POINT('Ctrl Pts',(0.0465809977751913,-0.0640886901070536,
0.033325));
#38246=CARTESIAN_POINT('Ctrl Pts',(0.0445852221789506,-0.0659878313900217,
0.033325));
#38247=CARTESIAN_POINT('Ctrl Pts',(0.0424886078928854,-0.0677910510833029,
0.033325));
#38248=CARTESIAN_POINT('Ctrl Pts',(0.0403143005657056,-0.0694828159680428,
0.033325));
#38249=CARTESIAN_POINT('Ctrl Pts',(0.0349826512621487,-0.0736312162225759,
0.033325));
#38250=CARTESIAN_POINT('Ctrl Pts',(0.0291714649030019,-0.0771273603905254,
0.033325));
#38251=CARTESIAN_POINT('Ctrl Pts',(0.0230262842057801,-0.0798880535992034,
0.033325));
#38252=CARTESIAN_POINT('Ctrl Pts',(0.0208180884878706,-0.0808800750257857,
0.033325));
#38253=CARTESIAN_POINT('Ctrl Pts',(0.0185640638716545,-0.0817776312978301,
0.033325));
#38254=CARTESIAN_POINT('Ctrl Pts',(0.0162773829813682,-0.0825731145983514,
0.033325));
#38255=CARTESIAN_POINT('Ctrl Pts',(0.0121340440651408,-0.0840144862082949,
0.033325));
#38256=CARTESIAN_POINT('Ctrl Pts',(0.00789937518293787,-0.0851163747295676,
0.033325));
#38257=CARTESIAN_POINT('Ctrl Pts',(0.0036115325539914,-0.0858581761147571,
0.033325));
#38258=CARTESIAN_POINT('Ctrl Pts',(-0.00150101100008291,-0.0867426516467301,
0.033325));
#38259=CARTESIAN_POINT('Ctrl Pts',(-0.00668928069841552,-0.0871159893456262,
0.033325));
#38260=CARTESIAN_POINT('Ctrl Pts',(-0.0118965134956391,-0.0870119718507496,
0.033325));
#38261=CARTESIAN_POINT('Ctrl Pts',(-0.0145396045993167,-0.0869591745731857,
0.033325));
#38262=CARTESIAN_POINT('Ctrl Pts',(-0.0171896073044249,-0.0867825364379904,
0.033325));
#38263=CARTESIAN_POINT('Ctrl Pts',(-0.0198217339970555,-0.0864878592704142,
0.033325));
#38264=CARTESIAN_POINT('Ctrl Pts',(-0.0253481174327742,-0.0858691584220329,
0.033325));
#38265=CARTESIAN_POINT('Ctrl Pts',(-0.0308111441111724,-0.0847318941000841,
0.033325));
#38266=CARTESIAN_POINT('Ctrl Pts',(-0.0361443503728786,-0.0831174822393533,
0.033325));
#38267=CARTESIAN_POINT('Ctrl Pts',(-0.0403416519334237,-0.0818469194503115,
0.033325));
#38268=CARTESIAN_POINT('Ctrl Pts',(-0.0444588266991117,-0.0802804065246257,
0.033325));
#38269=CARTESIAN_POINT('Ctrl Pts',(-0.0484639623864034,-0.0784300134796681,
0.033325));
#38270=CARTESIAN_POINT('Ctrl Pts',(-0.0509415676276126,-0.0772853472649801,
0.033325));
#38271=CARTESIAN_POINT('Ctrl Pts',(-0.053367724951023,-0.076035724041335,
0.033325));
#38272=CARTESIAN_POINT('Ctrl Pts',(-0.055731883450712,-0.0746874037064015,
0.033325));
#38273=CARTESIAN_POINT('Ctrl Pts',(-0.0622516783351781,-0.0709690523253594,
0.033325));
#38274=CARTESIAN_POINT('Ctrl Pts',(-0.0683093364934852,-0.0664998270329524,
0.033325));
#38275=CARTESIAN_POINT('Ctrl Pts',(-0.0737521082015833,-0.061343066863607,
0.033325));
#38276=CARTESIAN_POINT('Ctrl Pts',(-0.0753068057249169,-0.0598700669485494,
0.033325));
#38277=CARTESIAN_POINT('Ctrl Pts',(-0.0768112297895693,-0.0583406634828853,
0.033325));
#38278=CARTESIAN_POINT('Ctrl Pts',(-0.0782614497120756,-0.0567556262758528,
0.033325));
#38279=CARTESIAN_POINT('Ctrl Pts',(0.0666656654670482,-0.0321318641035092,
0.033325));
#38280=CARTESIAN_POINT('Ctrl Pts',(0.0760414822059936,-0.0123520292445354,
0.0352169166056634));
#38281=CARTESIAN_POINT('Ctrl Pts',(0.0764671442019932,0.0388397324871015,
0.0392004890110805));
#38282=CARTESIAN_POINT('Ctrl Pts',(0.0123509105275246,0.0861162136430816,
0.0452757172162514));
#38283=CARTESIAN_POINT('Ctrl Pts',(-0.0582325826622868,0.0603173335870826,
0.0510026081428899));
#38284=CARTESIAN_POINT('Ctrl Pts',(-0.0737281452942561,0.0178630175061391,
0.0546378432697745));
#38285=CARTESIAN_POINT('Ctrl Pts',(-0.0738797477720541,-6.29004154842593E-5,
0.0561814225969054));
#38286=CARTESIAN_POINT('Origin',(-2.39206768658147E-17,-5.43753587379397E-18,
0.033325));
#38287=CARTESIAN_POINT('',(0.0518589764809551,0.0526484240822814,0.033325));
#38288=CARTESIAN_POINT('Ctrl Pts',(-0.0929447515460691,0.0270916053744145,
0.033325));
#38289=CARTESIAN_POINT('Ctrl Pts',(-0.0917896323636415,0.0298912877885352,
0.033325));
#38290=CARTESIAN_POINT('Ctrl Pts',(-0.0904976311659083,0.032627221089921,
0.0333249999999999));
#38291=CARTESIAN_POINT('Ctrl Pts',(-0.0890666151901405,0.0352888178066413,
0.0333249999999999));
#38292=CARTESIAN_POINT('Ctrl Pts',(-0.0864865082201888,0.0400876490959472,
0.033325));
#38293=CARTESIAN_POINT('Ctrl Pts',(-0.0834548326657697,0.0446455583417202,
0.033325));
#38294=CARTESIAN_POINT('Ctrl Pts',(-0.0800249269923783,0.0489205910950087,
0.033325));
#38295=CARTESIAN_POINT('Ctrl Pts',(-0.0781132858485567,0.051303259681428,
0.033325));
#38296=CARTESIAN_POINT('Ctrl Pts',(-0.0760836906850449,0.0535904891565725,
0.033325));
#38297=CARTESIAN_POINT('Ctrl Pts',(-0.0739470307071451,0.0557748355204373,
0.033325));
#38298=CARTESIAN_POINT('Ctrl Pts',(-0.0705067602284846,0.059291886613499,
0.033325));
#38299=CARTESIAN_POINT('Ctrl Pts',(-0.0667883681472276,0.0625435339072888,
0.033325));
#38300=CARTESIAN_POINT('Ctrl Pts',(-0.0628308692529389,0.0654950879562435,
0.033325));
#38301=CARTESIAN_POINT('Ctrl Pts',(-0.0606814402551841,0.0670981600052135,
0.033325));
#38302=CARTESIAN_POINT('Ctrl Pts',(-0.0584651587268817,0.0686094986793821,
0.033325));
#38303=CARTESIAN_POINT('Ctrl Pts',(-0.0561952079986995,0.0700200058301,
0.033325));
#38304=CARTESIAN_POINT('Ctrl Pts',(-0.0501333136738915,0.0737867595247431,
0.033325));
#38305=CARTESIAN_POINT('Ctrl Pts',(-0.0436751701263957,0.0768486853796021,
0.033325));
#38306=CARTESIAN_POINT('Ctrl Pts',(-0.0369436491597186,0.0790891055682764,
0.033325));
#38307=CARTESIAN_POINT('Ctrl Pts',(-0.0333356887224549,0.0802899259242701,
0.033325));
#38308=CARTESIAN_POINT('Ctrl Pts',(-0.0296423557823287,0.0812543742145633,
0.033325));
#38309=CARTESIAN_POINT('Ctrl Pts',(-0.0259190414490983,0.0819530919554474,
0.033325));
#38310=CARTESIAN_POINT('Ctrl Pts',(-0.0231274480643262,0.0824769627997288,
0.033325));
#38311=CARTESIAN_POINT('Ctrl Pts',(-0.0203161830499112,0.0828528623331501,
0.033325));
#38312=CARTESIAN_POINT('Ctrl Pts',(-0.0174934788191478,0.0830727961543361,
0.033325));
#38313=CARTESIAN_POINT('Ctrl Pts',(-0.0126601868498688,0.0834493869285754,
0.033325));
#38314=CARTESIAN_POINT('Ctrl Pts',(-0.00779291433087069,0.0833692530579157,
0.0333249999999999));
#38315=CARTESIAN_POINT('Ctrl Pts',(-0.00294800581945059,0.0828496701715294,
0.0333249999999999));
#38316=CARTESIAN_POINT('Ctrl Pts',(0.000101264618999113,0.0825226570335005,
0.0333249999999999));
#38317=CARTESIAN_POINT('Ctrl Pts',(0.00314435587318879,0.0820201134909955,
0.0333249999999999));
#38318=CARTESIAN_POINT('Ctrl Pts',(0.00614210873778604,0.0813512661027619,
0.0333249999999999));
#38319=CARTESIAN_POINT('Ctrl Pts',(0.0106275580743664,0.0803504894512721,
0.0333249999999999));
#38320=CARTESIAN_POINT('Ctrl Pts',(0.0150235960594789,0.0789773917259045,
0.0333249999999999));
#38321=CARTESIAN_POINT('Ctrl Pts',(0.0192810923841575,0.0772484640679705,
0.033325));
#38322=CARTESIAN_POINT('Ctrl Pts',(0.0225362012762144,0.0759265961522092,
0.033325));
#38323=CARTESIAN_POINT('Ctrl Pts',(0.0257102610124195,0.0743964750603324,
0.033325));
#38324=CARTESIAN_POINT('Ctrl Pts',(0.0287775749945677,0.0726622576048804,
0.033325));
#38325=CARTESIAN_POINT('Ctrl Pts',(0.0308073950195533,0.0715146250706033,
0.033325));
#38326=CARTESIAN_POINT('Ctrl Pts',(0.0327876490113005,0.0702787831601469,
0.033325));
#38327=CARTESIAN_POINT('Ctrl Pts',(0.0347028232812334,0.0689622789254883,
0.033325));
#38328=CARTESIAN_POINT('Ctrl Pts',(0.0397377314622753,0.0655012477047154,
0.033325));
#38329=CARTESIAN_POINT('Ctrl Pts',(0.0443444553862968,0.0614742134119748,
0.033325));
#38330=CARTESIAN_POINT('Ctrl Pts',(0.0483819446640243,0.0569075936409299,
0.033325));
#38331=CARTESIAN_POINT('Ctrl Pts',(0.0495941607609181,0.0555365113632898,
0.0333249999999999));
#38332=CARTESIAN_POINT('Ctrl Pts',(0.0507547452462496,0.0541166472553641,
0.033325));
#38333=CARTESIAN_POINT('Ctrl Pts',(0.051858976480955,0.0526484240822815,
0.033325));
#38334=CARTESIAN_POINT('Origin',(0.,0.,0.033325));
#38335=CARTESIAN_POINT('Origin',(0.,0.,-0.0517230892635719));
#38336=CARTESIAN_POINT('Ctrl Pts',(0.0518589764809551,0.0526484240822814,
0.033325));
#38337=CARTESIAN_POINT('Ctrl Pts',(0.034560993232641,0.0696870291702574,
0.0354166557997537));
#38338=CARTESIAN_POINT('Ctrl Pts',(-0.0178308073244973,0.085128264632029,
0.0395999673992612));
#38339=CARTESIAN_POINT('Ctrl Pts',(-0.0679537005351042,0.0429705670053581,
0.0445839376447373));
#38340=CARTESIAN_POINT('Ctrl Pts',(-0.0738777383652924,0.0093611306850835,
0.0474762520904596));
#38341=CARTESIAN_POINT('Ctrl Pts',(-0.0738258018559393,4.09328341953522E-5,
0.0482769107364281));
#38342=CARTESIAN_POINT('Ctrl Pts',(0.0678412253220073,0.0688739702050683,
0.0201758476192062));
#38343=CARTESIAN_POINT('Ctrl Pts',(0.045212233027951,0.0911636474294266,
0.02226750341896));
#38344=CARTESIAN_POINT('Ctrl Pts',(-0.0233260256846517,0.111363666891765,
0.0264508150184675));
#38345=CARTESIAN_POINT('Ctrl Pts',(-0.105880745319823,0.0419279921909746,
0.0327257824177288));
#38346=CARTESIAN_POINT('Ctrl Pts',(-0.0933501081980039,-0.0650449563313979,
0.0390007498169901));
#38347=CARTESIAN_POINT('Ctrl Pts',(0.00262407842631599,-0.113778593381263,
0.0452757172162514));
#38348=CARTESIAN_POINT('Ctrl Pts',(0.0963221634673791,-0.0606354881256659,
0.0515506846155127));
#38349=CARTESIAN_POINT('Ctrl Pts',(0.103735822611175,0.0467997517633499,
0.057825652014774));
#38350=CARTESIAN_POINT('Ctrl Pts',(0.0182857197834144,0.112331107839639,
0.0641006194140354));
#38351=CARTESIAN_POINT('Ctrl Pts',(-0.0835478711919389,0.0772822483167664,
0.0703755868132966));
#38352=CARTESIAN_POINT('Ctrl Pts',(-0.11056795310426,-0.026964309214831,
0.076650554212558));
#38353=CARTESIAN_POINT('Ctrl Pts',(-0.0385895394868932,-0.107067331885508,
0.0829255216118192));
#38354=CARTESIAN_POINT('Ctrl Pts',(0.0679430878111881,-0.0913033084985679,
0.0892004890110805));
#38355=CARTESIAN_POINT('Ctrl Pts',(0.113639378289663,0.00621271467693868,
0.0954754564103418));
#38356=CARTESIAN_POINT('Ctrl Pts',(0.0575844881496173,0.0981660422492194,
0.101750423809603));
#38357=CARTESIAN_POINT('Ctrl Pts',(-0.0500310870203194,0.102222289415193,
0.108025391208864));
#38358=CARTESIAN_POINT('Ctrl Pts',(-0.112849420354528,0.0147501067708153,
0.114300358608126));
#38359=CARTESIAN_POINT('Ctrl Pts',(-0.0746231935625905,-0.0859298847748101,
0.120575326007387));
#38360=CARTESIAN_POINT('Ctrl Pts',(0.0304191741242974,-0.109667771340055,
0.126850293406648));
#38361=CARTESIAN_POINT('Ctrl Pts',(0.108225920969254,-0.0352128203351555,
0.13312526080591));
#38362=CARTESIAN_POINT('Ctrl Pts',(0.089125584578444,0.0707762354892434,
0.139400228205171));
#38363=CARTESIAN_POINT('Ctrl Pts',(-0.00977177477518579,0.113383641129007,
0.145675195604432));
#38364=CARTESIAN_POINT('Ctrl Pts',(-0.0999293420097319,0.0544862202834464,
0.151950163003694));
#38365=CARTESIAN_POINT('Ctrl Pts',(-0.100592616842759,-0.0532313773645962,
0.158225130402955));
#38366=CARTESIAN_POINT('Ctrl Pts',(-0.0112216609370024,-0.113221744247947,
0.164500097802216));
#38367=CARTESIAN_POINT('Ctrl Pts',(0.0882648350855844,-0.0719583743977188,
0.170775065201478));
#38368=CARTESIAN_POINT('Ctrl Pts',(0.108586899430732,0.0339831583264558,
0.177050032600739));
#38369=CARTESIAN_POINT('Ctrl Pts',(0.0575098468247979,0.0839498311266844,
0.181233344200246));
#38370=CARTESIAN_POINT('Ctrl Pts',(0.0270116869336335,0.0928246971123492,
0.183325));
#38371=CARTESIAN_POINT('Ctrl Pts',(0.0625138090416566,0.063465454830806,
0.0245588984128041));
#38372=CARTESIAN_POINT('Ctrl Pts',(0.0416618197628477,0.0840047746763702,
0.0266505542125579));
#38373=CARTESIAN_POINT('Ctrl Pts',(-0.0214942862312669,0.102618532805186,
0.0308338658120654));
#38374=CARTESIAN_POINT('Ctrl Pts',(-0.0975661725255505,0.0386354828481611,
0.0371088332113267));
#38375=CARTESIAN_POINT('Ctrl Pts',(-0.0860195376809465,-0.059937124660171,
0.043383800610588));
#38376=CARTESIAN_POINT('Ctrl Pts',(0.00241801554842842,-0.104843820640091,
0.0496587680098493));
#38377=CARTESIAN_POINT('Ctrl Pts',(0.0887582042467272,-0.0558739219087465,
0.0559337354091106));
#38378=CARTESIAN_POINT('Ctrl Pts',(0.095589685692049,0.0431246742824077,
0.062208702808372));
#38379=CARTESIAN_POINT('Ctrl Pts',(0.0168497840259201,0.103510002827837,
0.0684836702076332));
#38380=CARTESIAN_POINT('Ctrl Pts',(-0.0769870479305082,0.0712134500910467,
0.0747586376068947));
#38381=CARTESIAN_POINT('Ctrl Pts',(-0.101885304601719,-0.0248468636761093,
0.0810336050061557));
#38382=CARTESIAN_POINT('Ctrl Pts',(-0.0355591912003177,-0.0986595791618033,
0.0873085724054173));
#38383=CARTESIAN_POINT('Ctrl Pts',(0.0626076725025084,-0.0841334684811387,
0.0935835398046782));
#38384=CARTESIAN_POINT('Ctrl Pts',(0.104715537791268,0.00572484440104077,
0.0998585072039399));
#38385=CARTESIAN_POINT('Ctrl Pts',(0.0530625099835711,0.0904572874445442,
0.106133474603201));
#38386=CARTESIAN_POINT('Ctrl Pts',(-0.0461022601712969,0.0941950067966907,
0.112408442002462));
#38387=CARTESIAN_POINT('Ctrl Pts',(-0.103987613446247,0.0135918146177068,
0.118683409401724));
#38388=CARTESIAN_POINT('Ctrl Pts',(-0.0687632048257988,-0.0791820074340765,
0.124958376800985));
#38389=CARTESIAN_POINT('Ctrl Pts',(0.0280304259450684,-0.101055812052856,
0.131233344200246));
#38390=CARTESIAN_POINT('Ctrl Pts',(0.0997271868943474,-0.0324476380814423,
0.137508311599508));
#38391=CARTESIAN_POINT('Ctrl Pts',(0.0821267562402867,0.0652183395724518,
0.143783278998769));
#38392=CARTESIAN_POINT('Ctrl Pts',(-0.00900441964888684,0.104479883085,
0.15005824639803));
#38393=CARTESIAN_POINT('Ctrl Pts',(-0.0920821193073042,0.0502075420075893,
0.156333213797291));
#38394=CARTESIAN_POINT('Ctrl Pts',(-0.0926933086845182,-0.0490512390334914,
0.162608181196553));
#38395=CARTESIAN_POINT('Ctrl Pts',(-0.0103404495661197,-0.104330699595772,
0.168883148595814));
#38396=CARTESIAN_POINT('Ctrl Pts',(0.0813335994366777,-0.0663076478158446,
0.175158115995075));
#38397=CARTESIAN_POINT('Ctrl Pts',(0.100059818542758,0.0313145386182065,
0.181433083394337));
#38398=CARTESIAN_POINT('Ctrl Pts',(0.0529937300712946,0.0773574428708091,
0.185616394993844));
#38399=CARTESIAN_POINT('Ctrl Pts',(0.0248905209310009,0.0855353859263006,
0.187708050793598));
#38400=CARTESIAN_POINT('Ctrl Pts',(0.0571863927613058,0.0580569394565437,
0.028941949206402));
#38401=CARTESIAN_POINT('Ctrl Pts',(0.0381114064977443,0.0768459019233138,
0.0310336050061558));
#38402=CARTESIAN_POINT('Ctrl Pts',(-0.0196625467778821,0.0938733987186076,
0.0352169166056633));
#38403=CARTESIAN_POINT('Ctrl Pts',(-0.0892515997312777,0.0353429735053478,
0.0414918840049247));
#38404=CARTESIAN_POINT('Ctrl Pts',(-0.0786889671638893,-0.0548292929889441,
0.0477668514041859));
#38405=CARTESIAN_POINT('Ctrl Pts',(0.00221195267054096,-0.0959090478989199,
0.0540418188034473));
#38406=CARTESIAN_POINT('Ctrl Pts',(0.0811942450260753,-0.0511123556918271,
0.0603167862027086));
#38407=CARTESIAN_POINT('Ctrl Pts',(0.0874435487729231,0.0394495968014654,
0.0665917536019698));
#38408=CARTESIAN_POINT('Ctrl Pts',(0.0154138482684258,0.0946888978160358,
0.0728667210012312));
#38409=CARTESIAN_POINT('Ctrl Pts',(-0.0704262246690777,0.0651446518653269,
0.0791416884004924));
#38410=CARTESIAN_POINT('Ctrl Pts',(-0.0932026560991779,-0.0227294181373876,
0.0854166557997538));
#38411=CARTESIAN_POINT('Ctrl Pts',(-0.0325288429137424,-0.0902518264380986,
0.091691623199015));
#38412=CARTESIAN_POINT('Ctrl Pts',(0.0572722571938289,-0.0769636284637097,
0.0979665905982764));
#38413=CARTESIAN_POINT('Ctrl Pts',(0.0957916972928727,0.00523697412514306,
0.104241557997538));
#38414=CARTESIAN_POINT('Ctrl Pts',(0.0485405318175249,0.0827485326398688,
0.110516525396799));
#38415=CARTESIAN_POINT('Ctrl Pts',(-0.0421734333222743,0.0861677241781889,
0.11679149279606));
#38416=CARTESIAN_POINT('Ctrl Pts',(-0.0951258065379651,0.0124335224645981,
0.123066460195321));
#38417=CARTESIAN_POINT('Ctrl Pts',(-0.0629032160890072,-0.0724341300933428,
0.129341427594583));
#38418=CARTESIAN_POINT('Ctrl Pts',(0.0256416777658396,-0.092443852765658,
0.135616394993844));
#38419=CARTESIAN_POINT('Ctrl Pts',(0.0912284528194409,-0.029682455827729,
0.141891362393105));
#38420=CARTESIAN_POINT('Ctrl Pts',(0.0751279279021295,0.05966044365566,
0.148166329792367));
#38421=CARTESIAN_POINT('Ctrl Pts',(-0.00823706452258799,0.0955761250409928,
0.154441297191628));
#38422=CARTESIAN_POINT('Ctrl Pts',(-0.0842348966048762,0.0459288637317318,
0.160716264590889));
#38423=CARTESIAN_POINT('Ctrl Pts',(-0.0847940005262773,-0.0448711007023865,
0.166991231990151));
#38424=CARTESIAN_POINT('Ctrl Pts',(-0.00945923819523702,-0.0954396549435973,
0.173266199389412));
#38425=CARTESIAN_POINT('Ctrl Pts',(0.0744023637877709,-0.0606569212339703,
0.179541166788673));
#38426=CARTESIAN_POINT('Ctrl Pts',(0.0915327376547826,0.0286459189099571,
0.185816134187935));
#38427=CARTESIAN_POINT('Ctrl Pts',(0.0484776133177914,0.0707650546149338,
0.189999445787442));
#38428=CARTESIAN_POINT('Ctrl Pts',(0.0227693549283683,0.078246074740252,
0.192091101587196));
#38429=CARTESIAN_POINT('Ctrl Pts',(0.0518589764809551,0.0526484240822814,
0.033325));
#38430=CARTESIAN_POINT('Ctrl Pts',(0.034560993232641,0.0696870291702574,
0.0354166557997537));
#38431=CARTESIAN_POINT('Ctrl Pts',(-0.0178308073244973,0.085128264632029,
0.0395999673992612));
#38432=CARTESIAN_POINT('Ctrl Pts',(-0.0809370269370047,0.0320504641625344,
0.0458749347985226));
#38433=CARTESIAN_POINT('Ctrl Pts',(-0.071358396646832,-0.0497214613177173,
0.0521499021977838));
#38434=CARTESIAN_POINT('Ctrl Pts',(0.00200588979265343,-0.0869742751577483,
0.0584248695970452));
#38435=CARTESIAN_POINT('Ctrl Pts',(0.0736302858054235,-0.0463507894749077,
0.0646998369963064));
#38436=CARTESIAN_POINT('Ctrl Pts',(0.079297411853797,0.0357745193205231,
0.0709748043955678));
#38437=CARTESIAN_POINT('Ctrl Pts',(0.0139779125109316,0.0858677928042342,
0.077249771794829));
#38438=CARTESIAN_POINT('Ctrl Pts',(-0.0638654014076472,0.0590758536396072,
0.0835247391940904));
#38439=CARTESIAN_POINT('Ctrl Pts',(-0.0845200075966366,-0.0206119725986659,
0.0897997065933516));
#38440=CARTESIAN_POINT('Ctrl Pts',(-0.0294984946271671,-0.081844073714394,
0.0960746739926129));
#38441=CARTESIAN_POINT('Ctrl Pts',(0.0519368418851493,-0.0697937884462804,
0.102349641391874));
#38442=CARTESIAN_POINT('Ctrl Pts',(0.0868678567944775,0.00474910384924522,
0.108624608791136));
#38443=CARTESIAN_POINT('Ctrl Pts',(0.0440185536514787,0.0750397778351934,
0.114899576190397));
#38444=CARTESIAN_POINT('Ctrl Pts',(-0.0382446064732518,0.078140441559687,
0.121174543589658));
#38445=CARTESIAN_POINT('Ctrl Pts',(-0.0862639996296835,0.0112752303114895,
0.127449510988919));
#38446=CARTESIAN_POINT('Ctrl Pts',(-0.0570432273522154,-0.0656862527526091,
0.133724478388181));
#38447=CARTESIAN_POINT('Ctrl Pts',(0.0232529295866107,-0.0838318934784593,
0.139999445787442));
#38448=CARTESIAN_POINT('Ctrl Pts',(0.0827297187445345,-0.0269172735740158,
0.146274413186704));
#38449=CARTESIAN_POINT('Ctrl Pts',(0.0681290995639721,0.0541025477388684,
0.152549380585964));
#38450=CARTESIAN_POINT('Ctrl Pts',(-0.00746970939628905,0.0866723669969857,
0.158824347985226));
#38451=CARTESIAN_POINT('Ctrl Pts',(-0.0763876739024484,0.0416501854558747,
0.165099315384487));
#38452=CARTESIAN_POINT('Ctrl Pts',(-0.0768946923680362,-0.0406909623712818,
0.171374282783749));
#38453=CARTESIAN_POINT('Ctrl Pts',(-0.00857802682435435,-0.0865486102914224,
0.17764925018301));
#38454=CARTESIAN_POINT('Ctrl Pts',(0.0674711281388642,-0.0550061946520962,
0.183924217582271));
#38455=CARTESIAN_POINT('Ctrl Pts',(0.0830056567668076,0.0259772992017078,
0.190199184981532));
#38456=CARTESIAN_POINT('Ctrl Pts',(0.0439614965642881,0.0641726663590585,
0.19438249658104));
#38457=CARTESIAN_POINT('Ctrl Pts',(0.0206481889257357,0.0709567635542034,
0.196474152380794));
#38458=CARTESIAN_POINT('Ctrl Pts',(0.0270116869336335,0.0928246971123492,
0.183325));
#38459=CARTESIAN_POINT('Ctrl Pts',(0.0575098468247979,0.0839498311266844,
0.181233344200246));
#38460=CARTESIAN_POINT('Ctrl Pts',(0.083048373127765,0.0589664947265702,
0.179141688400492));
#38461=CARTESIAN_POINT('Ctrl Pts',(0.0924306255550574,0.0288179044058174,
0.177050032600739));
#38462=CARTESIAN_POINT('Ctrl Pts',(0.10181287798235,-0.00133068591493571,
0.174958376800985));
#38463=CARTESIAN_POINT('Ctrl Pts',(0.095038856533967,-0.0366445301563275,
0.172866721001231));
#38464=CARTESIAN_POINT('Ctrl Pts',(0.0750707631393444,-0.0611786805853946,
0.170775065201477));
#38465=CARTESIAN_POINT('Ctrl Pts',(0.055102669744722,-0.0857128310144614,
0.168683409401724));
#38466=CARTESIAN_POINT('Ctrl Pts',(0.02194050440386,-0.0994672876312039,
0.16659175360197));
#38467=CARTESIAN_POINT('Ctrl Pts',(-0.00953573758419697,-0.0963461214590169,
0.164500097802216));
#38468=CARTESIAN_POINT('Ctrl Pts',(-0.0410119795722545,-0.0932249552868299,
0.162408442002462));
#38469=CARTESIAN_POINT('Ctrl Pts',(-0.070802298207507,-0.073228166325713,
0.160316786202709));
#38470=CARTESIAN_POINT('Ctrl Pts',(-0.0855869117196286,-0.0452768389038139,
0.158225130402955));
#38471=CARTESIAN_POINT('Ctrl Pts',(-0.092884710370865,-0.0314798492569381,
0.157192673053848));
#38472=CARTESIAN_POINT('Ctrl Pts',(-0.0965263909752696,-0.0157447479797163,
0.156160215704741));
#38473=CARTESIAN_POINT('Ctrl Pts',(-0.0965227763075221,-6.77612820726425E-6,
0.155127758355634));
#38474=CARTESIAN_POINT('Origin',(0.,0.,0.1025));
#38475=CARTESIAN_POINT('Origin',(0.,0.,0.183325));
#38476=CARTESIAN_POINT('Origin',(0.,0.,0.0975096189432334));
#38477=CARTESIAN_POINT('',(0.,0.,0.0840192378864668));
#38478=CARTESIAN_POINT('',(-0.0400285208940887,4.90207999875487E-18,0.11));
#38479=CARTESIAN_POINT('',(-0.0207846096908265,-2.54538057293978E-18,0.0975096189432334));
#38480=CARTESIAN_POINT('Origin',(0.,0.,0.11));
#38481=CARTESIAN_POINT('Origin',(0.,0.0519615242270663,0.2));
#38482=CARTESIAN_POINT('',(3.18172571617472E-18,0.0519615242270663,0.2));
#38483=CARTESIAN_POINT('',(0.045,0.0259807621135332,0.2));
#38484=CARTESIAN_POINT('',(0.01125,0.045466333698683,0.2));
#38485=CARTESIAN_POINT('',(0.,0.0519615242270663,0.11));
#38486=CARTESIAN_POINT('',(3.18172571617472E-18,0.0519615242270663,0.2));
#38487=CARTESIAN_POINT('',(0.045,0.0259807621135332,0.11));
#38488=CARTESIAN_POINT('',(0.045,0.0259807621135332,0.11));
#38489=CARTESIAN_POINT('',(0.045,0.0259807621135332,0.2));
#38490=CARTESIAN_POINT('Origin',(-0.045,0.0259807621135332,0.2));
#38491=CARTESIAN_POINT('',(-0.045,0.0259807621135332,0.2));
#38492=CARTESIAN_POINT('',(-0.03375,0.0324759526419164,0.2));
#38493=CARTESIAN_POINT('',(-0.045,0.0259807621135332,0.11));
#38494=CARTESIAN_POINT('',(-0.045,0.0259807621135332,0.2));
#38495=CARTESIAN_POINT('',(3.18172571617472E-18,0.0519615242270663,0.11));
#38496=CARTESIAN_POINT('Origin',(-0.045,-0.0259807621135332,0.2));
#38497=CARTESIAN_POINT('',(-0.045,-0.0259807621135332,0.2));
#38498=CARTESIAN_POINT('',(-0.045,-0.0129903810567666,0.2));
#38499=CARTESIAN_POINT('',(-0.045,-0.0259807621135332,0.11));
#38500=CARTESIAN_POINT('',(-0.045,-0.0259807621135332,0.2));
#38501=CARTESIAN_POINT('',(-0.045,0.0259807621135332,0.11));
#38502=CARTESIAN_POINT('Origin',(-6.93889390390723E-18,-0.0519615242270663,
0.2));
#38503=CARTESIAN_POINT('',(-9.54517714852416E-18,-0.0519615242270663,0.2));
#38504=CARTESIAN_POINT('',(-0.01125,-0.045466333698683,0.2));
#38505=CARTESIAN_POINT('',(-6.93889390390723E-18,-0.0519615242270663,0.11));
#38506=CARTESIAN_POINT('',(-9.54517714852416E-18,-0.0519615242270663,0.2));
#38507=CARTESIAN_POINT('',(-0.045,-0.0259807621135332,0.11));
#38508=CARTESIAN_POINT('Origin',(0.045,-0.0259807621135332,0.2));
#38509=CARTESIAN_POINT('',(0.045,-0.0259807621135332,0.2));
#38510=CARTESIAN_POINT('',(0.03375,-0.0324759526419165,0.2));
#38511=CARTESIAN_POINT('',(0.045,-0.0259807621135332,0.11));
#38512=CARTESIAN_POINT('',(0.045,-0.0259807621135332,0.2));
#38513=CARTESIAN_POINT('',(-9.54517714852416E-18,-0.0519615242270663,0.11));
#38514=CARTESIAN_POINT('Origin',(0.045,0.0259807621135332,0.2));
#38515=CARTESIAN_POINT('',(0.045,0.0129903810567666,0.2));
#38516=CARTESIAN_POINT('',(0.045,-0.0259807621135332,0.11));
#38517=CARTESIAN_POINT('Origin',(0.,0.,0.11));
#38518=CARTESIAN_POINT('Origin',(0.07,0.,0.));
#38519=CARTESIAN_POINT('',(-0.07,-8.57252759403147E-18,8.67361737988404E-18));
#38520=CARTESIAN_POINT('Origin',(0.,0.,0.));
#38521=CARTESIAN_POINT('Origin',(0.,0.,0.0125));
#38522=CARTESIAN_POINT('',(-0.085,-1.04094977927525E-17,0.0125));
#38523=CARTESIAN_POINT('Origin',(0.,0.,0.19));
#38524=CARTESIAN_POINT('',(-0.08,-9.79717439317883E-18,0.2));
#38525=CARTESIAN_POINT('Origin',(0.,0.,0.2));
#38526=CARTESIAN_POINT('',(-0.09,-1.10218211923262E-17,0.19));
#38527=CARTESIAN_POINT('Origin',(0.,0.,0.2));
#54973=UNCERTAINTY_MEASURE_WITH_UNIT(LENGTH_MEASURE(0.001),#55003,
'DISTANCE_ACCURACY_VALUE',
'Maximum model space distance between geometric entities at asserted c
onnectivities');
#54980=UNCERTAINTY_MEASURE_WITH_UNIT(LENGTH_MEASURE(0.001),#55003,
'DISTANCE_ACCURACY_VALUE',
'Maximum model space distance between geometric entities at asserted c
onnectivities');
#54995=(
GEOMETRIC_REPRESENTATION_CONTEXT(3)
GLOBAL_UNCERTAINTY_ASSIGNED_CONTEXT((#54973))
GLOBAL_UNIT_ASSIGNED_CONTEXT((#55003,#55005,#55006))
REPRESENTATION_CONTEXT('','3D')
);
#55002=(
GEOMETRIC_REPRESENTATION_CONTEXT(3)
GLOBAL_UNCERTAINTY_ASSIGNED_CONTEXT((#54980))
GLOBAL_UNIT_ASSIGNED_CONTEXT((#55003,#55005,#55006))
REPRESENTATION_CONTEXT('','3D')
);
#55003=(
LENGTH_UNIT()
NAMED_UNIT(*)
SI_UNIT(.CENTI.,.METRE.)
);
#55005=(
NAMED_UNIT(*)
PLANE_ANGLE_UNIT()
SI_UNIT($,.RADIAN.)
);
#55006=(
NAMED_UNIT(*)
SI_UNIT($,.STERADIAN.)
SOLID_ANGLE_UNIT()
);
#55021=SHAPE_DEFINITION_REPRESENTATION(#55042,#55117);
#55042=PRODUCT_DEFINITION_SHAPE('',$,#55139);
#55117=SHAPE_REPRESENTATION('',(#26151),#54995);
#55124=PRODUCT_DEFINITION_CONTEXT('part definition',#55189,'design');
#55139=PRODUCT_DEFINITION('2026-10-18-23-37-08-575',
'20_ISO_4026_M2x2_Set_Screw',#55160,#55124);
#55160=PRODUCT_DEFINITION_FORMATION('',$,#55205);
#55189=APPLICATION_CONTEXT(
'Core Data for Automotive Mechanical Design Process');
#55190=PRODUCT_CONTEXT('part definition',#55189,'mechanical');
#55205=PRODUCT('2026-10-18-23-37-08-575','20_ISO_4026_M2x2_Set_Screw',$,
(#55190));
#55387=COLOUR_RGB('Black',0.12,0.14,0.17);
#55388=FILL_AREA_STYLE_COLOUR('',#55387);
#55389=FILL_AREA_STYLE('',(#55388));
#55390=SURFACE_STYLE_FILL_AREA(#55389);
#55391=SURFACE_SIDE_STYLE('',(#55390));
#55392=SURFACE_STYLE_USAGE(.BOTH.,#55391);
#55393=PRESENTATION_STYLE_ASSIGNMENT((#55392));
ENDSEC;
END-ISO-10303-21;
